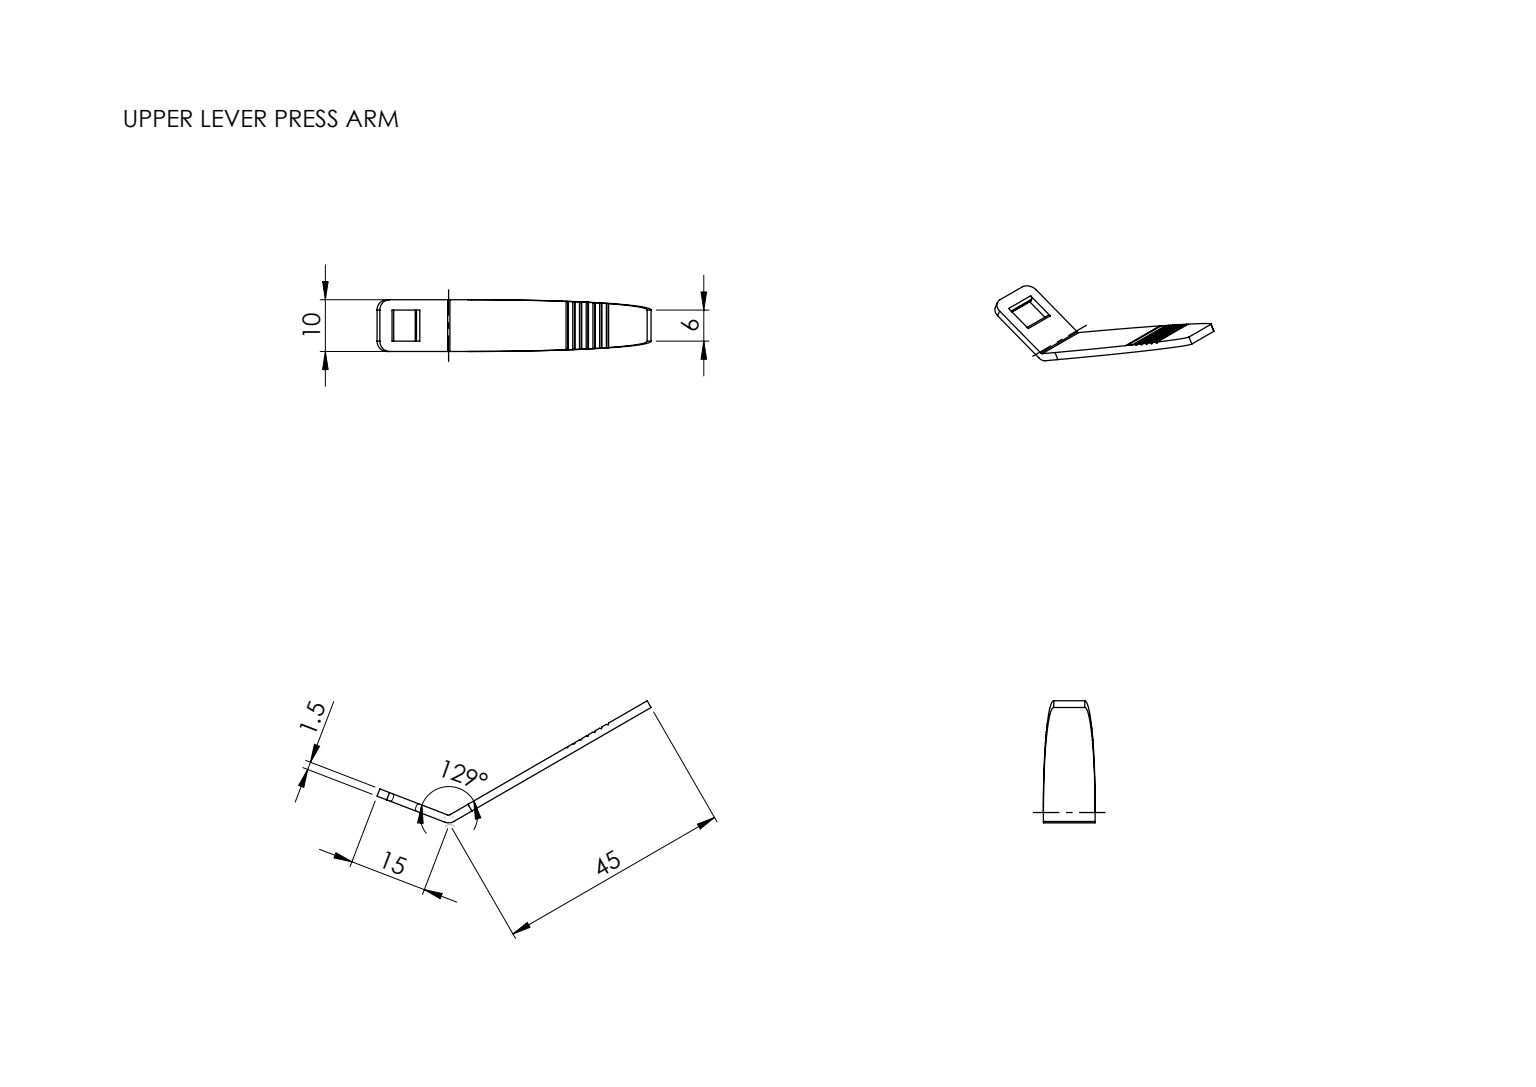
ISO-10303-21;
HEADER;
FILE_DESCRIPTION (('STEP AP214'),
    '1' );
FILE_NAME ('Upper Lever Press Arm.step',
    '2026-09-30T04:43:20',
    ( '' ),
    ( '' ),
    'SwSTEP 2.0',
    'SolidWorks 2026',
    '' );
FILE_SCHEMA (( 'AUTOMOTIVE_DESIGN' ));
ENDSEC;

DATA;
#3=B_SPLINE_CURVE_WITH_KNOTS ( 'NONE', 3,
 ( #22146, #34945, #44004, #5128 ),
 .UNSPECIFIED., .F., .F.,
 ( 4, 4 ),
 ( 1.885719144749635755E-05, 0.0003537736795864013565 ),
 .UNSPECIFIED. ) ;
#4=DIRECTION ( 'NONE',  ( 0.9659258262890682012, -0.2588190451025213501, 0.000000000000000000 ) ) ;
#132=CARTESIAN_POINT ( 'NONE',  ( -22.94165982901027689, 19.41290236794502277, -4.465504107374588472 ) ) ;
#193=CARTESIAN_POINT ( 'NONE',  ( -28.44450197225234334, 14.50378416766731959, -4.731833325462559969 ) ) ;
#237=LINE ( 'NONE', #8811, #24972 ) ;
#310=B_SPLINE_CURVE_WITH_KNOTS ( 'NONE', 3,
 ( #32716, #11134, #41787, #2878 ),
 .UNSPECIFIED., .F., .F.,
 ( 4, 4 ),
 ( 0.000000000000000000, 0.0003538863460372422966 ),
 .UNSPECIFIED. ) ;
#369=FACE_OUTER_BOUND ( 'NONE', #44588, .T. ) ;
#373=CARTESIAN_POINT ( 'NONE',  ( -27.13182931993292257, 16.99370688441070953, -4.657437592157545936 ) ) ;
#418=DIRECTION ( 'NONE',  ( -0.2588190451025176864, -0.9659258262890692004, 0.000000000000000000 ) ) ;
#455=EDGE_CURVE ( 'NONE', #37705, #6581, #56077, .T. ) ;
#460=VERTEX_POINT ( 'NONE', #2963 ) ;
#518=EDGE_CURVE ( 'NONE', #53934, #18987, #43004, .T. ) ;
#531=AXIS2_PLACEMENT_3D ( 'NONE', #51602, #12442, #13280 ) ;
#533=ADVANCED_FACE ( 'NONE', ( #51248 ), #3542, .F. ) ;
#534=AXIS2_PLACEMENT_3D ( 'NONE', #24826, #46384, #7499 ) ;
#571=AXIS2_PLACEMENT_3D ( 'NONE', #25411, #12058, #16909 ) ;
#582=( NAMED_UNIT ( * ) PLANE_ANGLE_UNIT ( ) SI_UNIT ( $, .RADIAN. ) );
#607=VERTEX_POINT ( 'NONE', #29699 ) ;
#614=ORIENTED_EDGE ( 'NONE', *, *, #13717, .F. ) ;
#616=VECTOR ( 'NONE', #50544, 1000.000000000000000 ) ;
#646=PLANE ( 'NONE',  #28564 ) ;
#675=DIRECTION ( 'NONE',  ( 0.2113248654051873565, 0.7886751345948123104, 0.5773502691896265082 ) ) ;
#682=VERTEX_POINT ( 'NONE', #21973 ) ;
#688=ORIENTED_EDGE ( 'NONE', *, *, #44373, .T. ) ;
#692=LINE ( 'NONE', #17737, #6878 ) ;
#697=CARTESIAN_POINT ( 'NONE',  ( -23.39689027546016220, 18.96061615304027370, 4.493364425890089109 ) ) ;
#727=EDGE_CURVE ( 'NONE', #44683, #32191, #692, .T. ) ;
#732=CARTESIAN_POINT ( 'NONE',  ( -16.70782865829815833, 23.01200647243835462, -4.019104856592038644 ) ) ;
#746=EDGE_CURVE ( 'NONE', #48518, #40704, #31739, .T. ) ;
#780=CARTESIAN_POINT ( 'NONE',  ( -20.79248460937205323, 18.92167845196996367, -4.386225263874957037 ) ) ;
#841=FILL_AREA_STYLE_COLOUR ( '', #31666 ) ;
#914=ORIENTED_EDGE ( 'NONE', *, *, #11163, .T. ) ;
#919=CARTESIAN_POINT ( 'NONE',  ( -50.99228148001754590, 2.341865487272627000, 5.000000000000000000 ) ) ;
#945=ORIENTED_EDGE ( 'NONE', *, *, #16723, .T. ) ;
#951=FILL_AREA_STYLE_COLOUR ( '', #1196 ) ;
#958=DIRECTION ( 'NONE',  ( 0.9335804264972041855, -0.3583679495452941621, 0.000000000000000000 ) ) ;
#963=EDGE_LOOP ( 'NONE', ( #48660, #54179, #26989, #34399, #45764, #5188, #19645, #55104, #36476, #32181 ) ) ;
#968=CARTESIAN_POINT ( 'NONE',  ( -21.06965149344186372, 20.49370688441071664, 4.356723378946029790 ) ) ;
#974=DIRECTION ( 'NONE',  ( 0.000000000000000000, 0.000000000000000000, 1.000000000000000000 ) ) ;
#985=CARTESIAN_POINT ( 'NONE',  ( -16.14528680376529834, 23.33679016358333769, -3.961395337094443914 ) ) ;
#1039=FACE_BOUND ( 'NONE', #10706, .T. ) ;
#1042=CARTESIAN_POINT ( 'NONE',  ( -28.39101450145270178, 14.53466517333176533, -4.730044803147324117 ) ) ;
#1050=CARTESIAN_POINT ( 'NONE',  ( -22.26155136248034694, 19.71499928042501537, 4.429874044484920503 ) ) ;
#1107=LINE ( 'NONE', #22455, #28687 ) ;
#1123=FACE_OUTER_BOUND ( 'NONE', #15703, .T. ) ;
#1180=ORIENTED_EDGE ( 'NONE', *, *, #37039, .T. ) ;
#1191=EDGE_LOOP ( 'NONE', ( #4345, #38872, #49783 ) ) ;
#1196=COLOUR_RGB ( '', 0.40784314, 0.44705882, 0.49803922) ;
#1254=DIRECTION ( 'NONE',  ( 0.9659258262890682012, -0.2588190451025213501, 0.000000000000000000 ) ) ;
#1307=LINE ( 'NONE', #53002, #19425 ) ;
#1330=CARTESIAN_POINT ( 'NONE',  ( -24.92324194630820244, 18.23204470015658174, -4.564397236248976419 ) ) ;
#1405=PRESENTATION_STYLE_ASSIGNMENT (( #23550 ) ) ;
#1409=CARTESIAN_POINT ( 'NONE',  ( -25.83279121425626812, 17.74370688441070953, -4.657437592157546824 ) ) ;
#1456=AXIS2_PLACEMENT_3D ( 'NONE', #26545, #39337, #35359 ) ;
#1459=DIRECTION ( 'NONE',  ( -0.9335804264972041855, 0.3583679495452941621, 0.000000000000000000 ) ) ;
#1498=AXIS2_PLACEMENT_3D ( 'NONE', #24554, #42170, #41870 ) ;
#1509=CIRCLE ( 'NONE', #36867, 0.5000000000000004441 ) ;
#1533=VECTOR ( 'NONE', #44302, 1000.000000000000114 ) ;
#1551=ORIENTED_EDGE ( 'NONE', *, *, #30791, .T. ) ;
#1552=EDGE_CURVE ( 'NONE', #19985, #6581, #39063, .T. ) ;
#1599=CARTESIAN_POINT ( 'NONE',  ( -27.56484202182514665, 16.74370688441070953, -4.657437592157546824 ) ) ;
#1634=CARTESIAN_POINT ( 'NONE',  ( -28.32679246876683266, 14.57174378119085389, 4.727889153708476400 ) ) ;
#1636=LINE ( 'NONE', #18963, #55409 ) ;
#1736=CARTESIAN_POINT ( 'NONE',  ( -56.02165185617580079, 5.343604887189308705, 2.999999999999993339 ) ) ;
#1741=B_SPLINE_CURVE_WITH_KNOTS ( 'NONE', 3,
 ( #23369, #39838, #22787, #52607 ),
 .UNSPECIFIED., .F., .F.,
 ( 4, 4 ),
 ( 0.0001251225081293656771, 0.0003537265380804738486 ),
 .UNSPECIFIED. ) ;
#1743=PLANE ( 'NONE',  #41578 ) ;
#1765=DIRECTION ( 'NONE',  ( -1.007958083594381669E-15, 3.869188571150967118E-16, -1.000000000000000000 ) ) ;
#1827=CARTESIAN_POINT ( 'NONE',  ( -20.11552963796318494, 21.04456939451101150, -4.294601649057681492 ) ) ;
#1840=CARTESIAN_POINT ( 'NONE',  ( -29.14071270714143935, 15.83387752003526394, 4.730034822273776030 ) ) ;
#1943=CARTESIAN_POINT ( 'NONE',  ( -11.88054826722768276, 25.79903810567671130, 3.000000000000000888 ) ) ;
#1988=CARTESIAN_POINT ( 'NONE',  ( -11.88054826722768276, 25.79903810567671130, 5.000000000000000000 ) ) ;
#2121=CARTESIAN_POINT ( 'NONE',  ( -29.26563357085082728, 15.76175442574525043, 4.734210823084358921 ) ) ;
#2142=VERTEX_POINT ( 'NONE', #17518 ) ;
#2186=ORIENTED_EDGE ( 'NONE', *, *, #25414, .T. ) ;
#2193=VECTOR ( 'NONE', #958, 999.9999999999998863 ) ;
#2213=CARTESIAN_POINT ( 'NONE',  ( -46.28406441860501985, 5.387676038879166462, 5.000000000000000000 ) ) ;
#2217=ORIENTED_EDGE ( 'NONE', *, *, #55126, .F. ) ;
#2296=PLANE ( 'NONE',  #21068 ) ;
#2410=DIRECTION ( 'NONE',  ( 0.3583679495452941066, 0.9335804264972041855, -0.000000000000000000 ) ) ;
#2412=CARTESIAN_POINT ( 'NONE',  ( -22.03063064900203827, 19.66612883677992585, 4.421226519471689542 ) ) ;
#2427=ORIENTED_EDGE ( 'NONE', *, *, #28275, .F. ) ;
#2432=AXIS2_PLACEMENT_3D ( 'NONE', #47385, #8496, #54174 ) ;
#2450=CARTESIAN_POINT ( 'NONE',  ( -27.13299098042555002, 16.99303619941258603, -4.657414165320978405 ) ) ;
#2462=CARTESIAN_POINT ( 'NONE',  ( -23.66772770479517618, 18.99370688441070953, -4.503111145262439052 ) ) ;
#2485=ORIENTED_EDGE ( 'NONE', *, *, #28912, .F. ) ;
#2568=FACE_OUTER_BOUND ( 'NONE', #32711, .T. ) ;
#2573=CARTESIAN_POINT ( 'NONE',  ( -58.57533928340691887, 0.08623575067603483912, 2.999999999999993339 ) ) ;
#2604=ORIENTED_EDGE ( 'NONE', *, *, #55126, .T. ) ;
#2610=AXIS2_PLACEMENT_3D ( 'NONE', #34638, #13373, #3697 ) ;
#2628=DIRECTION ( 'NONE',  ( -0.000000000000000000, -0.000000000000000000, 1.000000000000000000 ) ) ;
#2637=CARTESIAN_POINT ( 'NONE',  ( -22.02230666951336246, 19.67040017278726438, 4.420763615217817133 ) ) ;
#2683=EDGE_LOOP ( 'NONE', ( #55117, #19603, #53392, #16395 ) ) ;
#2686=ORIENTED_EDGE ( 'NONE', *, *, #5710, .F. ) ;
#2691=PLANE ( 'NONE',  #38679 ) ;
#2713=ORIENTED_EDGE ( 'NONE', *, *, #38351, .F. ) ;
#2763=CARTESIAN_POINT ( 'NONE',  ( -19.33760068587298164, 21.49370688441072019, 4.239878526350478793 ) ) ;
#2766=DIRECTION ( 'NONE',  ( 0.3535533905932738974, -0.6123724356957929160, -0.7071067811865487940 ) ) ;
#2785=EDGE_LOOP ( 'NONE', ( #40511, #29941, #51061 ) ) ;
#2800=( BOUNDED_SURFACE ( )  B_SPLINE_SURFACE ( 2, 3, ( 
 ( #15547, #23270, #2213, #41672 ),
 ( #28335, #15020, #45653, #32877 ),
 ( #27817, #11304, #28636, #40593 ) ),
 .UNSPECIFIED., .F., .F., .T. ) 
 B_SPLINE_SURFACE_WITH_KNOTS ( ( 3, 3 ),
 ( 4, 4 ),
 ( 0.000000000000000000, 1.000000000000000000 ),
 ( -0.001575000000000004998, 7.500000000001961749E-05 ),
 .UNSPECIFIED. ) 
 GEOMETRIC_REPRESENTATION_ITEM ( )  RATIONAL_B_SPLINE_SURFACE ( (
 ( 1.000000000000000000, 1.000000000000000000, 1.000000000000000000, 1.000000000000000000),
 ( 0.7071067811865475727, 0.7071067811865475727, 0.7071067811865484609, 0.7071067811865484609),
 ( 1.000000000000000000, 1.000000000000000000, 1.000000000000000000, 1.000000000000000000) ) ) 
 REPRESENTATION_ITEM ( '' )  SURFACE ( )  );
#2812=DIRECTION ( 'NONE',  ( 0.9659258262890692004, -0.2588190451025176864, 0.000000000000000000 ) ) ;
#2829=DIRECTION ( 'NONE',  ( 0.9335804264972041855, -0.3583679495452941066, 0.000000000000000000 ) ) ;
#2855=EDGE_CURVE ( 'NONE', #53976, #35993, #43666, .T. ) ;
#2878=CARTESIAN_POINT ( 'NONE',  ( -19.77061338776520216, 21.24370688441071664, -4.270683379717145733 ) ) ;
#2911=VERTEX_POINT ( 'NONE', #46208 ) ;
#2944=CARTESIAN_POINT ( 'NONE',  ( -46.00906441860537655, 4.911362066797487103, -5.000000000000000000 ) ) ;
#2963=CARTESIAN_POINT ( 'NONE',  ( -60.92294909528611413, 7.225036622302098976, 2.999999999999993339 ) ) ;
#3005=CARTESIAN_POINT ( 'NONE',  ( -23.66772770479517618, 18.99370688441070953, -4.657437592157546824 ) ) ;
#3035=B_SPLINE_CURVE_WITH_KNOTS ( 'NONE', 3,
 ( #45030, #32522, #1827, #23445, #5547, #44723, #19152, #41320, #36223, #23165, #36482 ),
 .UNSPECIFIED., .F., .F.,
 ( 4, 1, 1, 2, 2, 1, 4 ),
 ( 0.2333392773190904879, 0.2451180778799246229, 0.2480627780201330179, 0.2495351280902372015, 0.2502713031252893350, 0.2510074781603415239, 0.2568968784407584804 ),
 .UNSPECIFIED. ) ;
#3158=CARTESIAN_POINT ( 'NONE',  ( -63.00984630926863161, 1.788483511016180305, 2.999999999999993339 ) ) ;
#3275=ADVANCED_FACE ( 'NONE', ( #21789 ), #18361, .F. ) ;
#3318=CARTESIAN_POINT ( 'NONE',  ( -13.01064681732981398, 25.14657540356444088, -3.506683753893632183 ) ) ;
#3363=DIRECTION ( 'NONE',  ( -0.7886751345948130876, 0.2113248654051844977, 0.5773502691896263972 ) ) ;
#3375=DIRECTION ( 'NONE',  ( 0.9659258262890692004, -0.2588190451025176864, 0.000000000000000000 ) ) ;
#3426=ORIENTED_EDGE ( 'NONE', *, *, #37039, .F. ) ;
#3434=CARTESIAN_POINT ( 'NONE',  ( -22.02230563637845151, 19.67040402849924163, -4.420763475398227449 ) ) ;
#3449=B_SPLINE_CURVE_WITH_KNOTS ( 'NONE', 3,
 ( #47504, #55745, #16551, #4070 ),
 .UNSPECIFIED., .F., .F.,
 ( 4, 4 ),
 ( 0.0001648889278767292786, 0.0003345323828099543780 ),
 .UNSPECIFIED. ) ;
#3450=CARTESIAN_POINT ( 'NONE',  ( -21.93567689722629765, 19.99370688441071309, -4.657437592157546824 ) ) ;
#3452=CARTESIAN_POINT ( 'NONE',  ( -26.26580391614848864, 17.49370688441070953, -4.622528711259356271 ) ) ;
#3464=EDGE_LOOP ( 'NONE', ( #10205, #16971, #45019 ) ) ;
#3503=CARTESIAN_POINT ( 'NONE',  ( -60.88973930853472183, 7.404220597074750110, 2.999999999999993339 ) ) ;
#3513=VERTEX_POINT ( 'NONE', #55810 ) ;
#3528=CARTESIAN_POINT ( 'NONE',  ( -11.91804826722769128, 25.86399001096056338, -3.000000000000000000 ) ) ;
#3529=CYLINDRICAL_SURFACE ( 'NONE', #534, 0.5000000000000004441 ) ;
#3540=CARTESIAN_POINT ( 'NONE',  ( -13.18266667305592499, 23.31520888598613084, -3.678144203997483430 ) ) ;
#3542=PLANE ( 'NONE',  #47657 ) ;
#3622=DIRECTION ( 'NONE',  ( -0.000000000000000000, -0.000000000000000000, -1.000000000000000000 ) ) ;
#3675=CARTESIAN_POINT ( 'NONE',  ( -25.85160320928759248, 17.67349956316208193, 4.606045228336897779 ) ) ;
#3697=DIRECTION ( 'NONE',  ( 1.000000000000000000, 0.000000000000000000, 0.000000000000000000 ) ) ;
#3709=ORIENTED_EDGE ( 'NONE', *, *, #38832, .F. ) ;
#3718=EDGE_CURVE ( 'NONE', #18779, #46324, #15132, .T. ) ;
#3727=PLANE ( 'NONE',  #24862 ) ;
#3739=ORIENTED_EDGE ( 'NONE', *, *, #43733, .F. ) ;
#3749=PLANE ( 'NONE',  #37824 ) ;
#3752=VERTEX_POINT ( 'NONE', #14884 ) ;
#3823=DIRECTION ( 'NONE',  ( 0.9659258262890682012, -0.2588190451025213501, 0.000000000000000000 ) ) ;
#3848=CARTESIAN_POINT ( 'NONE',  ( -20.16419826038267260, 21.01647055225602401, 4.297939206181997207 ) ) ;
#3851=CARTESIAN_POINT ( 'NONE',  ( -22.02230563637845151, 19.67040402849924163, -4.420763475398227449 ) ) ;
#3858=CARTESIAN_POINT ( 'NONE',  ( -50.45472955569960760, 3.742236127018431890, 5.000000000000000000 ) ) ;
#3887=EDGE_LOOP ( 'NONE', ( #8947, #2217, #37332, #24607 ) ) ;
#3889=ORIENTED_EDGE ( 'NONE', *, *, #36503, .T. ) ;
#3924=LINE ( 'NONE', #52478, #14635 ) ;
#3952=AXIS2_PLACEMENT_3D ( 'NONE', #17630, #4, #38360 ) ;
#3976=ADVANCED_FACE ( 'NONE', ( #56031, #44080 ), #646, .T. ) ;
#3981=DIRECTION ( 'NONE',  ( 1.007958083594381472E-15, -3.869188571150966132E-16, 1.000000000000000000 ) ) ;
#4011=EDGE_LOOP ( 'NONE', ( #28267, #55445, #12491, #53597 ) ) ;
#4044=ORIENTED_EDGE ( 'NONE', *, *, #50823, .F. ) ;
#4066=ORIENTED_EDGE ( 'NONE', *, *, #49513, .F. ) ;
#4070=CARTESIAN_POINT ( 'NONE',  ( -23.29661890453421691, 19.01267837833611551, -4.488312987714206059 ) ) ;
#4092=VERTEX_POINT ( 'NONE', #3434 ) ;
#4123=PLANE ( 'NONE',  #571 ) ;
#4149=CARTESIAN_POINT ( 'NONE',  ( -22.65299646082626239, 19.57956224127125111, 4.449815307286153043 ) ) ;
#4195=ORIENTED_EDGE ( 'NONE', *, *, #45589, .T. ) ;
#4222=CARTESIAN_POINT ( 'NONE',  ( -21.06965149344186372, 20.49370688441071664, -4.356725136697556344 ) ) ;
#4233=CARTESIAN_POINT ( 'NONE',  ( -19.63965433603666710, 19.58726532061008641, 4.312915315567922292 ) ) ;
#4238=CARTESIAN_POINT ( 'NONE',  ( -61.10213307005876970, 6.758246409053502823, -3.000000000000006217 ) ) ;
#4300=AXIS2_PLACEMENT_3D ( 'NONE', #38438, #30777, #26785 ) ;
#4345=ORIENTED_EDGE ( 'NONE', *, *, #55262, .F. ) ;
#4354=CARTESIAN_POINT ( 'NONE',  ( -20.72814514249575168, 20.40220053346460460, -4.343046601173932153 ) ) ;
#4360=EDGE_LOOP ( 'NONE', ( #51718, #33979, #28900, #15955 ) ) ;
#4382=PLANE ( 'NONE',  #4300 ) ;
#4399=CARTESIAN_POINT ( 'NONE',  ( -15.36885972723471561, 22.05300973765551475, -3.958603441819915414 ) ) ;
#4487=CARTESIAN_POINT ( 'NONE',  ( -19.77061338776520216, 21.24370688441071664, -4.657437592157546824 ) ) ;
#4490=CARTESIAN_POINT ( 'NONE',  ( -19.70957090889394081, 19.54689896845012598, -4.317539206161682408 ) ) ;
#4495=VERTEX_POINT ( 'NONE', #37008 ) ;
#4496=CARTESIAN_POINT ( 'NONE',  ( -19.52344721837093999, 19.65435753127615470, 4.305181340342182139 ) ) ;
#4499=EDGE_CURVE ( 'NONE', #19187, #9690, #14862, .T. ) ;
#4529=ORIENTED_EDGE ( 'NONE', *, *, #8617, .F. ) ;
#4537=CARTESIAN_POINT ( 'NONE',  ( -62.23823698199103660, 6.658783344088820222, -3.000000000000000000 ) ) ;
#4543=EDGE_CURVE ( 'NONE', #19187, #51242, #19685, .T. ) ;
#4555=CARTESIAN_POINT ( 'NONE',  ( -24.53374897521541698, 18.49370927080960669, -4.545578601930409413 ) ) ;
#4628=ORIENTED_EDGE ( 'NONE', *, *, #18960, .F. ) ;
#4629=CARTESIAN_POINT ( 'NONE',  ( -56.66762604419704985, 5.055998648713356580, -3.000000000000007105 ) ) ;
#4630=CARTESIAN_POINT ( 'NONE',  ( -24.74851972188836058, 18.25476655873277920, 4.557895469182953185 ) ) ;
#4701=CARTESIAN_POINT ( 'NONE',  ( -22.04728230093569152, 19.65758605842115969, -4.422151119964278010 ) ) ;
#4708=CARTESIAN_POINT ( 'NONE',  ( -63.56784591066751489, 8.775889882925216767, 5.000000000000000000 ) ) ;
#4759=CARTESIAN_POINT ( 'NONE',  ( -19.95056665410288943, 19.40776001008019236, -4.333296610429257179 ) ) ;
#4791=ORIENTED_EDGE ( 'NONE', *, *, #38882, .F. ) ;
#4839=EDGE_CURVE ( 'NONE', #27103, #49013, #33304, .T. ) ;
#4852=EDGE_LOOP ( 'NONE', ( #39303, #3889, #32640 ) ) ;
#4945=ADVANCED_FACE ( 'NONE', ( #23385 ), #17999, .F. ) ;
#4973=DIRECTION ( 'NONE',  ( 0.9659258262890692004, -0.2588190451025176864, 0.000000000000000000 ) ) ;
#5001=( BOUNDED_CURVE ( )  B_SPLINE_CURVE ( 2, ( #41086, #22935, #10981 ),
 .UNSPECIFIED., .F., .F. ) 
 B_SPLINE_CURVE_WITH_KNOTS ( ( 3, 3 ),
 ( 0.6158339227882835276, 0.6249778499672641319 ),
 .UNSPECIFIED. ) 
 CURVE ( )  GEOMETRIC_REPRESENTATION_ITEM ( )  RATIONAL_B_SPLINE_CURVE ( ( 0.8614131787543850560, 0.8620336302495723579, 0.8627030601714029689 ) ) 
 REPRESENTATION_ITEM ( '' )  );
#5045=CIRCLE ( 'NONE', #15888, 0.5000000000000004441 ) ;
#5058=CARTESIAN_POINT ( 'NONE',  ( -37.15891100857655971, 9.472517764717013122, -4.937199669358084186 ) ) ;
#5085=VECTOR ( 'NONE', #43649, 1000.000000000000114 ) ;
#5086=EDGE_LOOP ( 'NONE', ( #37843, #20900, #27083, #46358, #51235, #17479, #25512 ) ) ;
#5115=FACE_OUTER_BOUND ( 'NONE', #17806, .T. ) ;
#5128=CARTESIAN_POINT ( 'NONE',  ( -21.93567466420777379, 19.99370817364452790, -4.408991681665293427 ) ) ;
#5188=ORIENTED_EDGE ( 'NONE', *, *, #50318, .T. ) ;
#5193=DIRECTION ( 'NONE',  ( -1.000000000000000000, 0.000000000000000000, 0.000000000000000000 ) ) ;
#5233=ADVANCED_FACE ( 'NONE', ( #46610 ), #3727, .F. ) ;
#5265=DIRECTION ( 'NONE',  ( -1.000000000000000000, 0.000000000000000000, 0.000000000000000000 ) ) ;
#5275=CARTESIAN_POINT ( 'NONE',  ( -56.20083583094844926, 4.876814673940706335, 2.999999999999993339 ) ) ;
#5307=CARTESIAN_POINT ( 'NONE',  ( -19.42910703681909368, 21.15220053346460816, -4.255330291692488665 ) ) ;
#5338=CARTESIAN_POINT ( 'NONE',  ( -19.68509517508318751, 19.56103003995438883, -4.315923200200658449 ) ) ;
#5382=ORIENTED_EDGE ( 'NONE', *, *, #29011, .T. ) ;
#5388=ORIENTED_EDGE ( 'NONE', *, *, #28680, .F. ) ;
#5398=( NAMED_UNIT ( * ) SI_UNIT ( $, .STERADIAN. ) SOLID_ANGLE_UNIT ( ) );
#5452=VECTOR ( 'NONE', #49321, 1000.000000000000114 ) ;
#5543=CARTESIAN_POINT ( 'NONE',  ( -14.23203706048740713, 24.44140541789180787, -3.724779944465314241 ) ) ;
#5547=CARTESIAN_POINT ( 'NONE',  ( -20.39013098992649020, 20.88602823003513365, -4.312947112340340006 ) ) ;
#5560=CARTESIAN_POINT ( 'NONE',  ( -38.30474801573077315, 10.54301926775796439, 4.960515765732081306 ) ) ;
#5561=ORIENTED_EDGE ( 'NONE', *, *, #53550, .F. ) ;
#5569=ORIENTED_EDGE ( 'NONE', *, *, #23443, .F. ) ;
#5591=ORIENTED_EDGE ( 'NONE', *, *, #52151, .F. ) ;
#5604=CARTESIAN_POINT ( 'NONE',  ( -45.77156441860526570, 4.499999999999973355, 5.000000000000000000 ) ) ;
#5663=( NAMED_UNIT ( * ) SI_UNIT ( $, .STERADIAN. ) SOLID_ANGLE_UNIT ( ) );
#5695=EDGE_CURVE ( 'NONE', #35896, #40396, #13626, .T. ) ;
#5696=VECTOR ( 'NONE', #40835, 1000.000000000000000 ) ;
#5710=EDGE_CURVE ( 'NONE', #35896, #41243, #40512, .T. ) ;
#5711=EDGE_CURVE ( 'NONE', #54087, #19187, #10399, .T. ) ;
#5730=VECTOR ( 'NONE', #40205, 1000.000000000000000 ) ;
#5732=CARTESIAN_POINT ( 'NONE',  ( -50.02554558092695913, 3.776013638374817294, 5.000000000000000000 ) ) ;
#5807=DIRECTION ( 'NONE',  ( 0.3535533905932752297, -0.6123724356957952475, -0.7071067811865462405 ) ) ;
#5809=VECTOR ( 'NONE', #41899, 1000.000000000000000 ) ;
#5816=CARTESIAN_POINT ( 'NONE',  ( -27.13299098042555002, 16.99303619941258603, -4.657414165320978405 ) ) ;
#5838=CARTESIAN_POINT ( 'NONE',  ( -13.83440620147302269, 24.67097770138186874, -3.662372917584403087 ) ) ;
#5862=ORIENTED_EDGE ( 'NONE', *, *, #37251, .T. ) ;
#5864=ORIENTED_EDGE ( 'NONE', *, *, #50563, .T. ) ;
#5918=VERTEX_POINT ( 'NONE', #6685 ) ;
#5926=EDGE_CURVE ( 'NONE', #18779, #21631, #8828, .T. ) ;
#5927=CARTESIAN_POINT ( 'NONE',  ( -56.38001980572109062, 4.410024460692103077, -3.000000000000007105 ) ) ;
#5949=CARTESIAN_POINT ( 'NONE',  ( -61.38973930853472183, 7.404220597074748333, 2.999999999999993339 ) ) ;
#5959=CARTESIAN_POINT ( 'NONE',  ( -20.72814514249575168, 20.40220053346460460, 4.343046601168861542 ) ) ;
#5964=LINE ( 'NONE', #49096, #29767 ) ;
#5968=( NAMED_UNIT ( * ) PLANE_ANGLE_UNIT ( ) SI_UNIT ( $, .RADIAN. ) );
#5976=CIRCLE ( 'NONE', #11382, 0.5000000000000004441 ) ;
#5983=VECTOR ( 'NONE', #42987, 1000.000000000000000 ) ;
#6085=CARTESIAN_POINT ( 'NONE',  ( -50.27554558092695913, 4.209026340267034705, 5.000000000000000000 ) ) ;
#6091=DIRECTION ( 'NONE',  ( -0.000000000000000000, -0.000000000000000000, 1.000000000000000000 ) ) ;
#6101=CARTESIAN_POINT ( 'NONE',  ( -21.06965149344186372, 20.49370688441071664, -4.657437592157546824 ) ) ;
#6116=CARTESIAN_POINT ( 'NONE',  ( -61.21055533376208757, 7.871010810323348039, -3.000000000000007105 ) ) ;
#6117=ORIENTED_EDGE ( 'NONE', *, *, #50563, .F. ) ;
#6154=CARTESIAN_POINT ( 'NONE',  ( -30.55480944230645690, 15.01744838932757276, 4.775844711708173485 ) ) ;
#6263=B_SPLINE_CURVE_WITH_KNOTS ( 'NONE', 3,
 ( #10723, #10967, #1330, #28286 ),
 .UNSPECIFIED., .F., .F.,
 ( 4, 4 ),
 ( 0.0002184642560491729404, 0.0003536952807433174899 ),
 .UNSPECIFIED. ) ;
#6321=ADVANCED_FACE ( 'NONE', ( #8876 ), #21359, .T. ) ;
#6376=DIRECTION ( 'NONE',  ( -0.9335804264972041855, 0.3583679495452941621, 0.000000000000000000 ) ) ;
#6432=PRODUCT_DEFINITION_CONTEXT ( 'detailed design', #56163, 'design' ) ;
#6435=CARTESIAN_POINT ( 'NONE',  ( -44.89558674184503673, 6.737796755050466935, -5.000000000000005329 ) ) ;
#6494=PLANE ( 'NONE',  #45542 ) ;
#6505=CARTESIAN_POINT ( 'NONE',  ( -11.38054826722768098, 24.93301270189227381, 3.000000000000000000 ) ) ;
#6535=ORIENTED_EDGE ( 'NONE', *, *, #19165, .T. ) ;
#6580=ORIENTED_EDGE ( 'NONE', *, *, #52151, .T. ) ;
#6581=VERTEX_POINT ( 'NONE', #19313 ) ;
#6589=CARTESIAN_POINT ( 'NONE',  ( -19.42910703681909368, 21.15220053346460816, 4.255330291687501543 ) ) ;
#6683=EDGE_LOOP ( 'NONE', ( #33292, #29988, #10668, #9770 ) ) ;
#6685=CARTESIAN_POINT ( 'NONE',  ( -61.74810725808002587, 6.470640170577546257, -3.000000000000007105 ) ) ;
#6689=ORIENTED_EDGE ( 'NONE', *, *, #33111, .T. ) ;
#6723=ORIENTED_EDGE ( 'NONE', *, *, #19766, .F. ) ;
#6817=AXIS2_PLACEMENT_3D ( 'NONE', #16793, #12546, #20187 ) ;
#6825=VERTEX_POINT ( 'NONE', #39738 ) ;
#6832=ORIENTED_EDGE ( 'NONE', *, *, #727, .T. ) ;
#6857=ADVANCED_FACE ( 'NONE', ( #9915 ), #31196, .T. ) ;
#6878=VECTOR ( 'NONE', #31053, 1000.000000000000114 ) ;
#6887=CARTESIAN_POINT ( 'NONE',  ( -19.36810218178846910, 21.37987375194729367, 4.244941833917287077 ) ) ;
#6896=DIRECTION ( 'NONE',  ( -0.000000000000000000, -0.000000000000000000, 1.000000000000000000 ) ) ;
#7026=AXIS2_PLACEMENT_3D ( 'NONE', #8681, #20618, #43325 ) ;
#7058=AXIS2_PLACEMENT_3D ( 'NONE', #5732, #13433, #18217 ) ;
#7154=EDGE_CURVE ( 'NONE', #21504, #10403, #14203, .T. ) ;
#7177=ORIENTED_EDGE ( 'NONE', *, *, #11568, .F. ) ;
#7189=CARTESIAN_POINT ( 'NONE',  ( -26.26580391614848864, 17.49370688441070953, -4.657437592157546824 ) ) ;
#7222=ORIENTED_EDGE ( 'NONE', *, *, #55454, .T. ) ;
#7274=VERTEX_POINT ( 'NONE', #42088 ) ;
#7283=CARTESIAN_POINT ( 'NONE',  ( -22.02230666951336246, 19.67040017278726438, 4.420763615217817133 ) ) ;
#7361=AXIS2_PLACEMENT_3D ( 'NONE', #26935, #51898, #13017 ) ;
#7388=CARTESIAN_POINT ( 'NONE',  ( -11.88054826722768276, 25.79903810567671130, -3.000000000000000000 ) ) ;
#7435=ORIENTED_EDGE ( 'NONE', *, *, #7154, .F. ) ;
#7444=EDGE_CURVE ( 'NONE', #6825, #29855, #42683, .T. ) ;
#7499=DIRECTION ( 'NONE',  ( 1.000000000000000000, 0.000000000000000000, -8.673617379884027583E-16 ) ) ;
#7555=CARTESIAN_POINT ( 'NONE',  ( -20.53083501583961734, 20.80479272279814040, 4.322231945293713906 ) ) ;
#7556=CARTESIAN_POINT ( 'NONE',  ( -26.24927669643210848, 17.48927842923457021, -4.622014950999592031 ) ) ;
#7561=CARTESIAN_POINT ( 'NONE',  ( -13.00144731260268038, 25.15188674009506542, -3.504651694023052766 ) ) ;
#7567=DIRECTION ( 'NONE',  ( -0.9335804264972042965, 0.3583679495452938291, -0.000000000000000000 ) ) ;
#7592=CARTESIAN_POINT ( 'NONE',  ( -24.96676581047183063, 18.24370688441070953, -4.565775476651154463 ) ) ;
#7604=CARTESIAN_POINT ( 'NONE',  ( -23.44005680416443838, 18.93270265044663603, 4.490773887887535842 ) ) ;
#7659=VERTEX_POINT ( 'NONE', #14520 ) ;
#7677=DIRECTION ( 'NONE',  ( 0.000000000000000000, 0.000000000000000000, 1.000000000000000000 ) ) ;
#7729=B_SPLINE_CURVE_WITH_KNOTS ( 'NONE', 3,
 ( #49222, #10335, #27661, #44987 ),
 .UNSPECIFIED., .F., .F.,
 ( 4, 4 ),
 ( 0.7012410636449952772, 0.7288427234739881522 ),
 .UNSPECIFIED. ) ;
#7832=CARTESIAN_POINT ( 'NONE',  ( -19.42910703681909368, 21.15220053346460816, 4.255330291687501543 ) ) ;
#7915=LINE ( 'NONE', #7604, #47445 ) ;
#8073=LINE ( 'NONE', #16876, #21275 ) ;
#8135=CARTESIAN_POINT ( 'NONE',  ( -11.88054826722768276, 25.79903810567671130, -3.000000000000000000 ) ) ;
#8172=DIRECTION ( 'NONE',  ( -1.000000000000000000, 0.000000000000000000, 0.000000000000000000 ) ) ;
#8256=DIRECTION ( 'NONE',  ( 0.000000000000000000, 0.000000000000000000, -1.000000000000000000 ) ) ;
#8266=ORIENTED_EDGE ( 'NONE', *, *, #44650, .T. ) ;
#8284=ORIENTED_EDGE ( 'NONE', *, *, #40489, .T. ) ;
#8296=B_SPLINE_CURVE_WITH_KNOTS ( 'NONE', 3,
 ( #11566, #28883, #46181, #7283 ),
 .UNSPECIFIED., .F., .F.,
 ( 4, 4 ),
 ( 0.000000000000000000, 0.0003349204823136315776 ),
 .UNSPECIFIED. ) ;
#8325=EDGE_LOOP ( 'NONE', ( #15393, #45057, #35257, #5569 ) ) ;
#8375=FACE_OUTER_BOUND ( 'NONE', #29807, .T. ) ;
#8466=CARTESIAN_POINT ( 'NONE',  ( -19.36956794502930634, 19.74319977116263303, 4.294846203288412489 ) ) ;
#8496=DIRECTION ( 'NONE',  ( 0.9659258262890682012, -0.2588190451025213501, 0.000000000000000000 ) ) ;
#8504=CARTESIAN_POINT ( 'NONE',  ( -49.27554558092695913, 2.476975532698160620, 5.000000000000000000 ) ) ;
#8555=EDGE_LOOP ( 'NONE', ( #54942, #44710, #47319, #46606, #24688, #25642, #25519, #9963, #53675, #22278, #47759, #29937, #5388, #20429, #42126, #40703, #32041, #55171, #55584, #5591, #31627, #32561, #27281, #4628, #12436, #50794, #27262 ) ) ;
#8563=ORIENTED_EDGE ( 'NONE', *, *, #21234, .F. ) ;
#8564=ORIENTED_EDGE ( 'NONE', *, *, #50679, .F. ) ;
#8612=LINE ( 'NONE', #25944, #18397 ) ;
#8617=EDGE_CURVE ( 'NONE', #29855, #9917, #27180, .T. ) ;
#8642=CARTESIAN_POINT ( 'NONE',  ( -25.83279121425626812, 17.74370688441070953, 4.657440554554202805 ) ) ;
#8658=CARTESIAN_POINT ( 'NONE',  ( -13.19204130227259952, 23.30979644128433748, -3.679643887444146610 ) ) ;
#8674=EDGE_CURVE ( 'NONE', #50858, #45180, #46535, .T. ) ;
#8681=CARTESIAN_POINT ( 'NONE',  ( -62.23823698199103660, 6.658783344088824663, 3.000000000000000000 ) ) ;
#8706=CARTESIAN_POINT ( 'NONE',  ( -22.65298538027628794, 19.57956863862976249, -4.449819841089008854 ) ) ;
#8797=ORIENTED_EDGE ( 'NONE', *, *, #45589, .F. ) ;
#8811=CARTESIAN_POINT ( 'NONE',  ( -19.33760068587298164, 21.49370688441072019, -4.657437592157546824 ) ) ;
#8818=AXIS2_PLACEMENT_3D ( 'NONE', #16839, #43691, #35213 ) ;
#8819=CARTESIAN_POINT ( 'NONE',  ( -25.85160320928759248, 17.67349956316208193, 4.606045228336897779 ) ) ;
#8821=VECTOR ( 'NONE', #31799, 1000.000000000000000 ) ;
#8828=B_SPLINE_CURVE_WITH_KNOTS ( 'NONE', 3,
 ( #45864, #37071, #54372, #34757 ),
 .UNSPECIFIED., .F., .F.,
 ( 4, 4 ),
 ( 0.6233793831165909127, 0.6485820559972910182 ),
 .UNSPECIFIED. ) ;
#8876=FACE_OUTER_BOUND ( 'NONE', #32982, .T. ) ;
#8905=CARTESIAN_POINT ( 'NONE',  ( -26.21622229497770817, 17.48042152905857449, -4.621141326338904065 ) ) ;
#8927=DIRECTION ( 'NONE',  ( 0.8660254037844380415, 0.5000000000000011102, 0.000000000000000000 ) ) ;
#8928=ORIENTED_EDGE ( 'NONE', *, *, #29439, .T. ) ;
#8940=ORIENTED_EDGE ( 'NONE', *, *, #18960, .T. ) ;
#8941=CARTESIAN_POINT ( 'NONE',  ( -12.68893542602017988, 23.60026475436954740, -3.594889907554657427 ) ) ;
#8943=EDGE_LOOP ( 'NONE', ( #40478, #26337, #29664, #33700 ) ) ;
#8947=ORIENTED_EDGE ( 'NONE', *, *, #37432, .T. ) ;
#8963=ORIENTED_EDGE ( 'NONE', *, *, #33272, .T. ) ;
#8965=CARTESIAN_POINT ( 'NONE',  ( -56.20083583094844926, 4.876814673940706335, 2.999999999999993339 ) ) ;
#8969=CARTESIAN_POINT ( 'NONE',  ( -64.10539783498545319, 7.375519243179410545, 3.000000000000000000 ) ) ;
#8982=CARTESIAN_POINT ( 'NONE',  ( -45.77156441860526570, 4.499999999999973355, 5.000000000000000000 ) ) ;
#8983=CARTESIAN_POINT ( 'NONE',  ( -13.01702680972596227, 25.14289191323709360, -3.508089884283071669 ) ) ;
#8990=ORIENTED_EDGE ( 'NONE', *, *, #37009, .T. ) ;
#8991=CARTESIAN_POINT ( 'NONE',  ( -21.64218843024125860, 20.16315252982854034, -4.391944182239861050 ) ) ;
#8999=ORIENTED_EDGE ( 'NONE', *, *, #26082, .F. ) ;
#9021=DIRECTION ( 'NONE',  ( 0.000000000000000000, 0.000000000000000000, 1.000000000000000000 ) ) ;
#9051=ORIENTED_EDGE ( 'NONE', *, *, #19766, .T. ) ;
#9063=CARTESIAN_POINT ( 'NONE',  ( -50.27554558092695913, 4.209026340267034705, 5.000000000000000000 ) ) ;
#9082=CARTESIAN_POINT ( 'NONE',  ( -61.56892328330737030, 6.937430383826147740, 2.999999999999993339 ) ) ;
#9084=DIRECTION ( 'NONE',  ( 0.3535533905932738974, -0.6123724356957929160, -0.7071067811865487940 ) ) ;
#9115=CARTESIAN_POINT ( 'NONE',  ( -27.56460882755735398, 16.74384151918395247, 4.673983433494172779 ) ) ;
#9143=FACE_OUTER_BOUND ( 'NONE', #13193, .T. ) ;
#9171=CARTESIAN_POINT ( 'NONE',  ( -11.63054826722768453, 25.36602540378449788, -3.000000000000000000 ) ) ;
#9175=ORIENTED_EDGE ( 'NONE', *, *, #53550, .T. ) ;
#9224=CARTESIAN_POINT ( 'NONE',  ( -56.38001980572109062, 4.410024460692103077, 2.999999999999993339 ) ) ;
#9261=EDGE_LOOP ( 'NONE', ( #17584, #13863, #22718 ) ) ;
#9293=CARTESIAN_POINT ( 'NONE',  ( -37.09365488523594223, 9.510193405093987806, -4.936228699513737439 ) ) ;
#9299=CARTESIAN_POINT ( 'NONE',  ( -22.15441416008502529, 19.68629195356385964, 4.426028523006688253 ) ) ;
#9355=DIRECTION ( 'NONE',  ( 0.000000000000000000, 0.000000000000000000, 1.000000000000000000 ) ) ;
#9368=LINE ( 'NONE', #1409, #1533 ) ;
#9390=EDGE_LOOP ( 'NONE', ( #55400, #29866, #42316, #11635 ) ) ;
#9421=AXIS2_PLACEMENT_3D ( 'NONE', #23266, #27812, #32602 ) ;
#9426=DIRECTION ( 'NONE',  ( -0.7886751345948130876, 0.2113248654051844977, 0.5773502691896263972 ) ) ;
#9440=AXIS2_PLACEMENT_3D ( 'NONE', #51668, #7677, #38323 ) ;
#9510=CARTESIAN_POINT ( 'NONE',  ( -50.27554558092695913, 4.209026340267034705, 5.000000000000000000 ) ) ;
#9540=CARTESIAN_POINT ( 'NONE',  ( -15.35417357620467449, 23.79353959847493272, -3.874970200383425656 ) ) ;
#9565=B_SPLINE_CURVE_WITH_KNOTS ( 'NONE', 3,
 ( #16217, #12537, #21326, #12238 ),
 .UNSPECIFIED., .F., .F.,
 ( 4, 4 ),
 ( 0.000000000000000000, 0.0001352353904500101485 ),
 .UNSPECIFIED. ) ;
#9597=CARTESIAN_POINT ( 'NONE',  ( -50.45472955569960760, 3.742236127018431890, 5.000000000000000000 ) ) ;
#9600=CARTESIAN_POINT ( 'NONE',  ( -37.11431328563478615, 9.498266272062682702, -4.936536869034685360 ) ) ;
#9661=VECTOR ( 'NONE', #55067, 1000.000000000000114 ) ;
#9665=CARTESIAN_POINT ( 'NONE',  ( -20.63663879154963965, 20.74370688441071664, 4.329123301634322907 ) ) ;
#9673=CARTESIAN_POINT ( 'NONE',  ( -60.88973930853472183, 7.404220597074748333, 2.999999999999993339 ) ) ;
#9690=VERTEX_POINT ( 'NONE', #10975 ) ;
#9719=CARTESIAN_POINT ( 'NONE',  ( -24.57312748012714820, 18.34675972927921350, -4.549864808573585329 ) ) ;
#9741=DIRECTION ( 'NONE',  ( -1.000000000000000000, 0.000000000000000000, 0.000000000000000000 ) ) ;
#9747=ORIENTED_EDGE ( 'NONE', *, *, #32751, .T. ) ;
#9770=ORIENTED_EDGE ( 'NONE', *, *, #25414, .F. ) ;
#9773=EDGE_CURVE ( 'NONE', #31783, #27675, #1636, .T. ) ;
#9781=B_SPLINE_CURVE_WITH_KNOTS ( 'NONE', 3,
 ( #47430, #30413, #30699, #13628 ),
 .UNSPECIFIED., .F., .F.,
 ( 4, 4 ),
 ( 0.0001144323540671334324, 0.0003537324766284092063 ),
 .UNSPECIFIED. ) ;
#9795=CARTESIAN_POINT ( 'NONE',  ( -23.44701637808619665, 18.93456746265863799, 4.495868649597294819 ) ) ;
#9812=ORIENTED_EDGE ( 'NONE', *, *, #5926, .F. ) ;
#9859=EDGE_CURVE ( 'NONE', #32191, #49975, #53954, .T. ) ;
#9860=DIRECTION ( 'NONE',  ( 0.3535533905932738974, -0.6123724356957929160, 0.7071067811865487940 ) ) ;
#9868=CARTESIAN_POINT ( 'NONE',  ( -23.23471500290295921, 19.24370688441070953, 4.480778704491060971 ) ) ;
#9879=CARTESIAN_POINT ( 'NONE',  ( -38.32071399784587840, 8.801750496117048073, -4.953405659155169616 ) ) ;
#9915=FACE_OUTER_BOUND ( 'NONE', #51533, .T. ) ;
#9917=VERTEX_POINT ( 'NONE', #26555 ) ;
#9963=ORIENTED_EDGE ( 'NONE', *, *, #8674, .F. ) ;
#10058=EDGE_LOOP ( 'NONE', ( #48399, #39670, #10894, #44445 ) ) ;
#10085=CARTESIAN_POINT ( 'NONE',  ( -16.11986972353830083, 23.35146472169441267, -3.958709963775913554 ) ) ;
#10106=EDGE_LOOP ( 'NONE', ( #40506, #9747, #37023, #14379, #39036, #25268, #20038, #29547 ) ) ;
#10186=CARTESIAN_POINT ( 'NONE',  ( -25.54041736840764187, 17.91250900301538351, 4.591768117563441720 ) ) ;
#10197=CARTESIAN_POINT ( 'NONE',  ( -56.02165185617580079, 5.343604887189308705, 2.999999999999993339 ) ) ;
#10205=ORIENTED_EDGE ( 'NONE', *, *, #727, .F. ) ;
#10288=ORIENTED_EDGE ( 'NONE', *, *, #28680, .T. ) ;
#10303=ADVANCED_FACE ( 'NONE', ( #45833 ), #24268, .F. ) ;
#10308=EDGE_CURVE ( 'NONE', #48202, #45033, #46372, .T. ) ;
#10314=DIRECTION ( 'NONE',  ( 1.000000000000000000, 0.000000000000000000, -0.000000000000000000 ) ) ;
#10335=CARTESIAN_POINT ( 'NONE',  ( -21.64220182007004212, 20.16314479920728431, 4.391939828907996279 ) ) ;
#10356=CARTESIAN_POINT ( 'NONE',  ( -26.26580391614848864, 17.49370688441070953, -4.622528711259356271 ) ) ;
#10397=ORIENTED_EDGE ( 'NONE', *, *, #15013, .T. ) ;
#10399=LINE ( 'NONE', #1599, #34752 ) ;
#10403=VERTEX_POINT ( 'NONE', #25958 ) ;
#10460=EDGE_LOOP ( 'NONE', ( #20475, #13328, #28049 ) ) ;
#10469=EDGE_CURVE ( 'NONE', #44458, #50858, #1741, .T. ) ;
#10569=DIRECTION ( 'NONE',  ( -0.000000000000000000, -0.000000000000000000, -1.000000000000000000 ) ) ;
#10584=CARTESIAN_POINT ( 'NONE',  ( -24.96676581047183063, 18.24370688441070953, -4.657437592157546824 ) ) ;
#10614=ADVANCED_FACE ( 'NONE', ( #17015 ), #55074, .F. ) ;
#10653=VECTOR ( 'NONE', #42681, 1000.000000000000000 ) ;
#10668=ORIENTED_EDGE ( 'NONE', *, *, #44636, .F. ) ;
#10688=VERTEX_POINT ( 'NONE', #35729 ) ;
#10696=CARTESIAN_POINT ( 'NONE',  ( -19.33759994122731385, 21.49370731433205250, -4.239680377485293583 ) ) ;
#10706=EDGE_LOOP ( 'NONE', ( #45349, #39990, #19819, #15141 ) ) ;
#10723=CARTESIAN_POINT ( 'NONE',  ( -24.83619454210204580, 18.20872041849631984, -4.561852789702152577 ) ) ;
#10829=EDGE_CURVE ( 'NONE', #54076, #45033, #21954, .T. ) ;
#10849=CARTESIAN_POINT ( 'NONE',  ( -24.53374897521541698, 18.49370927080960669, -4.545578601930409413 ) ) ;
#10894=ORIENTED_EDGE ( 'NONE', *, *, #18197, .F. ) ;
#10936=CARTESIAN_POINT ( 'NONE',  ( -29.00661482377690703, 15.91129896909354180, 4.725528206980505352 ) ) ;
#10938=ORIENTED_EDGE ( 'NONE', *, *, #23443, .T. ) ;
#10948=CARTESIAN_POINT ( 'NONE',  ( -63.00984630926863161, 1.788483511016180305, 2.999999999999993339 ) ) ;
#10957=CARTESIAN_POINT ( 'NONE',  ( -29.02628690221330388, 15.89994128931277295, -4.726187803958536549 ) ) ;
#10967=CARTESIAN_POINT ( 'NONE',  ( -24.87971818958798309, 18.22038254469182661, -4.563127009718482618 ) ) ;
#10975=CARTESIAN_POINT ( 'NONE',  ( -27.13299098042555002, 16.99303619941258603, -4.657414165320978405 ) ) ;
#10981=CARTESIAN_POINT ( 'NONE',  ( -27.56460882755735753, 16.74384151918395247, 4.673983433494172779 ) ) ;
#11013=FACE_OUTER_BOUND ( 'NONE', #20075, .T. ) ;
#11046=VECTOR ( 'NONE', #18242, 1000.000000000000000 ) ;
#11088=DIRECTION ( 'NONE',  ( 0.3583679495452941066, 0.9335804264972041855, 0.000000000000000000 ) ) ;
#11092=CARTESIAN_POINT ( 'NONE',  ( -23.44701637808619665, 18.93456746265863799, 4.495868649597294819 ) ) ;
#11093=EDGE_CURVE ( 'NONE', #12998, #21622, #26288, .T. ) ;
#11134=CARTESIAN_POINT ( 'NONE',  ( -19.54294029912376729, 21.18270206417094315, -4.260498045023555669 ) ) ;
#11138=ORIENTED_EDGE ( 'NONE', *, *, #41766, .F. ) ;
#11163=EDGE_CURVE ( 'NONE', #34812, #49013, #3035, .T. ) ;
#11184=VECTOR ( 'NONE', #36642, 1000.000000000000000 ) ;
#11238=CARTESIAN_POINT ( 'NONE',  ( -37.63793934321780199, 10.92800143433129456, -4.933120776947167663 ) ) ;
#11260=CIRCLE ( 'NONE', #9440, 0.5000000000000004441 ) ;
#11295=ORIENTED_EDGE ( 'NONE', *, *, #10308, .T. ) ;
#11304=CARTESIAN_POINT ( 'NONE',  ( -11.36804826722768702, 24.91136206679766829, 3.000000000000000000 ) ) ;
#11317=CARTESIAN_POINT ( 'NONE',  ( -24.53375310857961367, 18.49370688441070953, 4.545578210335888159 ) ) ;
#11325=LINE ( 'NONE', #15311, #15717 ) ;
#11377=DIRECTION ( 'NONE',  ( 0.5000000000000011102, -0.8660254037844380415, 0.000000000000000000 ) ) ;
#11382=AXIS2_PLACEMENT_3D ( 'NONE', #6085, #23389, #40705 ) ;
#11412=LINE ( 'NONE', #3450, #17540 ) ;
#11435=ADVANCED_FACE ( 'NONE', ( #52613 ), #4382, .F. ) ;
#11479=ADVANCED_FACE ( 'NONE', ( #369 ), #43812, .F. ) ;
#11529=FACE_OUTER_BOUND ( 'NONE', #4360, .T. ) ;
#11537=CARTESIAN_POINT ( 'NONE',  ( -29.06878564040112067, 15.87540463137980851, -4.727619564647471684 ) ) ;
#11552=VERTEX_POINT ( 'NONE', #23086 ) ;
#11566=CARTESIAN_POINT ( 'NONE',  ( -21.93567689722629765, 19.99370688441071309, 4.408989160011352659 ) ) ;
#11568=EDGE_CURVE ( 'NONE', #2911, #38353, #22537, .T. ) ;
#11612=VERTEX_POINT ( 'NONE', #17905 ) ;
#11635=ORIENTED_EDGE ( 'NONE', *, *, #50425, .T. ) ;
#11660=PLANE ( 'NONE',  #24024 ) ;
#11712=LINE ( 'NONE', #15673, #32230 ) ;
#11745=ADVANCED_FACE ( 'NONE', ( #44549 ), #14471, .F. ) ;
#11752=DIRECTION ( 'NONE',  ( 0.8660254037844380415, 0.5000000000000011102, 0.000000000000000000 ) ) ;
#11762=CARTESIAN_POINT ( 'NONE',  ( -46.55906441860520317, 5.863990010960497656, -5.000000000000000000 ) ) ;
#11786=CARTESIAN_POINT ( 'NONE',  ( -26.03813301551774728, 17.43270265044663603, 4.490773887887535842 ) ) ;
#11819=B_SPLINE_CURVE_WITH_KNOTS ( 'NONE', 3,
 ( #4701, #34519, #43346, #3851 ),
 .UNSPECIFIED., .F., .F.,
 ( 4, 4 ),
 ( 0.0002388585478777321643, 0.0002669665482816597568 ),
 .UNSPECIFIED. ) ;
#11908=CARTESIAN_POINT ( 'NONE',  ( -26.25138199253913385, 17.50203338588876179, 4.621929860192643069 ) ) ;
#11965=LINE ( 'NONE', #50870, #22209 ) ;
#11988=DIRECTION ( 'NONE',  ( 1.007958083594381472E-15, -3.869188571150965146E-16, 1.000000000000000000 ) ) ;
#12018=DIRECTION ( 'NONE',  ( 0.2113248654051873565, 0.7886751345948123104, 0.5773502691896265082 ) ) ;
#12055=CARTESIAN_POINT ( 'NONE',  ( -19.65677579747983472, 21.21320419402555402, 4.265613255886147925 ) ) ;
#12058=DIRECTION ( 'NONE',  ( 0.5000000000000011102, -0.8660254037844380415, 0.000000000000000000 ) ) ;
#12156=FACE_OUTER_BOUND ( 'NONE', #39852, .T. ) ;
#12160=LINE ( 'NONE', #29495, #53719 ) ;
#12161=CARTESIAN_POINT ( 'NONE',  ( -19.66742376178725493, 19.57123263517775769, 4.314754536491465231 ) ) ;
#12172=CARTESIAN_POINT ( 'NONE',  ( -50.27554558092695913, 4.209026340267034705, 5.000000000000000000 ) ) ;
#12188=LINE ( 'NONE', #47110, #616 ) ;
#12220=CARTESIAN_POINT ( 'NONE',  ( -46.27156441860557123, 5.366025403784241199, -5.000000000000000000 ) ) ;
#12232=CARTESIAN_POINT ( 'NONE',  ( -22.04728230093569152, 19.65758605842115969, -4.422151119964278010 ) ) ;
#12238=CARTESIAN_POINT ( 'NONE',  ( -24.83619032682412353, 18.20871928901600256, 4.561852666301203563 ) ) ;
#12263=AXIS2_PLACEMENT_3D ( 'NONE', #9082, #9355, #36071 ) ;
#12289=AXIS2_PLACEMENT_3D ( 'NONE', #17929, #22472, #44029 ) ;
#12341=EDGE_CURVE ( 'NONE', #34812, #24159, #18096, .T. ) ;
#12348=CARTESIAN_POINT ( 'NONE',  ( -11.64304826722768382, 25.38767603887911051, -3.000000000000000000 ) ) ;
#12363=CARTESIAN_POINT ( 'NONE',  ( -12.29957260759845106, 23.82506348239776273, -3.515194272803603415 ) ) ;
#12384=VECTOR ( 'NONE', #6896, 1000.000000000000000 ) ;
#12436=ORIENTED_EDGE ( 'NONE', *, *, #15634, .F. ) ;
#12442=DIRECTION ( 'NONE',  ( 0.3535533905932752297, -0.6123724356957952475, -0.7071067811865462405 ) ) ;
#12491=ORIENTED_EDGE ( 'NONE', *, *, #19403, .F. ) ;
#12515=EDGE_CURVE ( 'NONE', #42394, #52748, #6263, .T. ) ;
#12516=B_SPLINE_CURVE_WITH_KNOTS ( 'NONE', 3,
 ( #44984, #31363, #697, #9795 ),
 .UNSPECIFIED., .F., .F.,
 ( 4, 4 ),
 ( 0.0001724778598249929792, 0.0003421153678589267371 ),
 .UNSPECIFIED. ) ;
#12537=CARTESIAN_POINT ( 'NONE',  ( -24.92324054119748311, 18.23204432365830030, 4.564397195367118520 ) ) ;
#12546=DIRECTION ( 'NONE',  ( 0.9659258262890682012, -0.2588190451025213501, 0.000000000000000000 ) ) ;
#12577=FACE_OUTER_BOUND ( 'NONE', #50426, .T. ) ;
#12661=CARTESIAN_POINT ( 'NONE',  ( -22.94167088982010583, 19.41289598198349253, 4.465499946586994895 ) ) ;
#12681=VERTEX_POINT ( 'NONE', #8969 ) ;
#12684=VERTEX_POINT ( 'NONE', #9224 ) ;
#12753=FACE_OUTER_BOUND ( 'NONE', #23953, .T. ) ;
#12794=LINE ( 'NONE', #30117, #15507 ) ;
#12836=EDGE_CURVE ( 'NONE', #25142, #26953, #35635, .T. ) ;
#12965=EDGE_LOOP ( 'NONE', ( #22878, #54116, #33746, #54474, #19413, #6689 ) ) ;
#12987=EDGE_CURVE ( 'NONE', #29855, #15218, #50367, .T. ) ;
#12998=VERTEX_POINT ( 'NONE', #54342 ) ;
#13017=DIRECTION ( 'NONE',  ( -1.000000000000000000, 0.000000000000000000, 0.000000000000000000 ) ) ;
#13099=EDGE_CURVE ( 'NONE', #44683, #48518, #9368, .T. ) ;
#13160=CLOSED_SHELL ( 'NONE', ( #43827, #29227, #10303, #44606, #53124, #11479, #44827, #54797, #35461, #17663, #28041, #14786, #3976, #6857, #17209, #55333, #11745, #53873, #10614, #49999, #27367, #4945, #44545, #11435, #47399, #6321, #54230, #41877, #33767, #22103, #3275, #22660, #54366, #49968, #45435, #15902, #44436, #51617, #34084, #56080, #5233, #36232, #18692, #53536, #533, #22020, #21448, #26237, #52711, #21500, #27690, #14677, #18516, #18199, #50674 ) ) ;
#13193=EDGE_LOOP ( 'NONE', ( #52620, #48064, #37638, #53051 ) ) ;
#13220=DIRECTION ( 'NONE',  ( 0.000000000000000000, 0.000000000000000000, 1.000000000000000000 ) ) ;
#13242=CARTESIAN_POINT ( 'NONE',  ( -46.02156441860523017, 4.933012701892206309, 5.000000000000000000 ) ) ;
#13280=DIRECTION ( 'NONE',  ( 0.3535533905932738974, -0.6123724356957929160, 0.7071067811865487940 ) ) ;
#13287=AXIS2_PLACEMENT_3D ( 'NONE', #22467, #31244, #14764 ) ;
#13288=CARTESIAN_POINT ( 'NONE',  ( -50.27554558092695913, 4.209026340267034705, 5.000000000000000000 ) ) ;
#13302=AXIS2_PLACEMENT_3D ( 'NONE', #12172, #16160, #20707 ) ;
#13304=CARTESIAN_POINT ( 'NONE',  ( -37.69457521496538277, 9.163251890963174162, -4.944930165255981613 ) ) ;
#13307=DIRECTION ( 'NONE',  ( -0.8660254037844379305, -0.5000000000000011102, 0.000000000000000000 ) ) ;
#13310=ORIENTED_EDGE ( 'NONE', *, *, #51462, .T. ) ;
#13328=ORIENTED_EDGE ( 'NONE', *, *, #33811, .T. ) ;
#13366=CARTESIAN_POINT ( 'NONE',  ( -50.45472955569960760, 3.742236127018431890, 5.000000000000000000 ) ) ;
#13373=DIRECTION ( 'NONE',  ( 0.000000000000000000, 0.000000000000000000, 1.000000000000000000 ) ) ;
#13390=APPLICATION_CONTEXT ( 'automotive_design' ) ;
#13433=DIRECTION ( 'NONE',  ( 0.5000000000000011102, -0.8660254037844380415, 0.000000000000000000 ) ) ;
#13452=CARTESIAN_POINT ( 'NONE',  ( -11.38054826722768276, 24.93301270189227736, -3.000000000000000000 ) ) ;
#13492=EDGE_CURVE ( 'NONE', #7274, #30542, #40027, .T. ) ;
#13505=CARTESIAN_POINT ( 'NONE',  ( -61.10213307005877681, 6.758246409053505488, -3.000000000000007105 ) ) ;
#13515=CARTESIAN_POINT ( 'NONE',  ( -13.57018763683711349, 24.82352436079930769, -3.618365315326378173 ) ) ;
#13517=B_SPLINE_CURVE_WITH_KNOTS ( 'NONE', 3,
 ( #36701, #6887, #49490, #6589 ),
 .UNSPECIFIED., .F., .F.,
 ( 4, 4 ),
 ( 0.000000000000000000, 0.0003539001916872983413 ),
 .UNSPECIFIED. ) ;
#13565=CARTESIAN_POINT ( 'NONE',  ( -19.68185725454445034, 19.56289945424903109, -4.315709269779091528 ) ) ;
#13574=PRODUCT_DEFINITION_FORMATION_WITH_SPECIFIED_SOURCE ( 'ANY', '', #31892, .NOT_KNOWN. ) ;
#13575=DIRECTION ( 'NONE',  ( 0.000000000000000000, 0.000000000000000000, 1.000000000000000000 ) ) ;
#13607=CARTESIAN_POINT ( 'NONE',  ( -25.25174164940481347, 18.07917600709017947, 4.578957096563475382 ) ) ;
#13626=B_SPLINE_CURVE_WITH_KNOTS ( 'NONE', 3,
 ( #5307, #22618, #14105, #10696 ),
 .UNSPECIFIED., .F., .F.,
 ( 4, 4 ),
 ( 0.000000000000000000, 0.0003539001916874550085 ),
 .UNSPECIFIED. ) ;
#13628=CARTESIAN_POINT ( 'NONE',  ( -23.23471098716119698, 19.24370920290025566, -4.480780584866845828 ) ) ;
#13696=AXIS2_PLACEMENT_3D ( 'NONE', #41721, #54499, #2812 ) ;
#13717=EDGE_CURVE ( 'NONE', #43487, #24159, #54742, .T. ) ;
#13725=ORIENTED_EDGE ( 'NONE', *, *, #39119, .T. ) ;
#13778=LINE ( 'NONE', #22328, #52275 ) ;
#13833=CARTESIAN_POINT ( 'NONE',  ( -15.40229489717257394, 22.03370593329148264, -3.962133388944282686 ) ) ;
#13857=ORIENTED_EDGE ( 'NONE', *, *, #44373, .F. ) ;
#13863=ORIENTED_EDGE ( 'NONE', *, *, #33593, .T. ) ;
#13937=ORIENTED_EDGE ( 'NONE', *, *, #34493, .F. ) ;
#13942=LINE ( 'NONE', #48876, #32736 ) ;
#13968=CARTESIAN_POINT ( 'NONE',  ( -22.02718324817240969, 19.65220053346460460, 4.407440554554201917 ) ) ;
#13980=EDGE_CURVE ( 'NONE', #24541, #2142, #55450, .T. ) ;
#14093=VERTEX_POINT ( 'NONE', #16283 ) ;
#14105=CARTESIAN_POINT ( 'NONE',  ( -19.36810218178845489, 21.37987375194732209, -4.244941833920536922 ) ) ;
#14115=VECTOR ( 'NONE', #54871, 1000.000000000000000 ) ;
#14140=CARTESIAN_POINT ( 'NONE',  ( -20.22851404498383587, 19.24728700913452073, -4.351128180092163511 ) ) ;
#14147=B_SPLINE_CURVE_WITH_KNOTS ( 'NONE', 3,
 ( #8982, #13242, #18311, #22023 ),
 .UNSPECIFIED., .F., .F.,
 ( 4, 4 ),
 ( 0.000000000000000000, 1.000000000000000000 ),
 .UNSPECIFIED. ) ;
#14199=DIRECTION ( 'NONE',  ( 0.9659258262890692004, -0.2588190451025176864, 0.000000000000000000 ) ) ;
#14203=B_SPLINE_CURVE_WITH_KNOTS ( 'NONE', 3,
 ( #27946, #44982, #49520, #27097 ),
 .UNSPECIFIED., .F., .F.,
 ( 4, 4 ),
 ( 0.7664662348551912752, 1.000000000000000000 ),
 .UNSPECIFIED. ) ;
#14220=SURFACE_SIDE_STYLE ('',( #31532 ) ) ;
#14284=DIRECTION ( 'NONE',  ( -0.2588190451025176864, -0.9659258262890692004, 0.000000000000000000 ) ) ;
#14291=EDGE_CURVE ( 'NONE', #46324, #40047, #20253, .T. ) ;
#14347=CARTESIAN_POINT ( 'NONE',  ( -22.36868959911851462, 19.74370688441071309, -4.657437592157546824 ) ) ;
#14369=CARTESIAN_POINT ( 'NONE',  ( -13.93117922710646539, 24.61510576898210445, -3.677906343404563572 ) ) ;
#14379=ORIENTED_EDGE ( 'NONE', *, *, #30791, .F. ) ;
#14385=CARTESIAN_POINT ( 'NONE',  ( -27.99202758151029613, 16.49707118653253346, 4.690121163682637651 ) ) ;
#14395=ORIENTED_EDGE ( 'NONE', *, *, #55203, .F. ) ;
#14428=CARTESIAN_POINT ( 'NONE',  ( -28.19207438693690904, 14.64952330200006259, 4.723338118696758237 ) ) ;
#14471=PLANE ( 'NONE',  #38622 ) ;
#14475=DIRECTION ( 'NONE',  ( -0.5000000000000015543, 0.8660254037844378194, 0.000000000000000000 ) ) ;
#14517=CARTESIAN_POINT ( 'NONE',  ( -50.45472955569960760, 3.742236127018431890, -5.000000000000000000 ) ) ;
#14520=CARTESIAN_POINT ( 'NONE',  ( -61.70068505767310540, 8.059153983834628221, -5.000000000000000000 ) ) ;
#14552=EDGE_CURVE ( 'NONE', #53976, #19985, #24884, .T. ) ;
#14561=CARTESIAN_POINT ( 'NONE',  ( -61.21055533376208047, 7.871010810323351592, 5.000000000000012434 ) ) ;
#14635=VECTOR ( 'NONE', #13575, 1000.000000000000000 ) ;
#14656=CARTESIAN_POINT ( 'NONE',  ( -46.52156441860571334, 5.799038105676371124, -5.000000000000000000 ) ) ;
#14677=ADVANCED_FACE ( 'NONE', ( #29856 ), #39502, .T. ) ;
#14764=DIRECTION ( 'NONE',  ( -0.3583679495452925523, -0.9335804264972047406, 0.000000000000000000 ) ) ;
#14786=ADVANCED_FACE ( 'NONE', ( #1123 ), #40326, .T. ) ;
#14862=LINE ( 'NONE', #27940, #14993 ) ;
#14884=CARTESIAN_POINT ( 'NONE',  ( -45.77156441860525149, 4.499999999999981348, -5.000000000000000000 ) ) ;
#14921=VECTOR ( 'NONE', #9021, 1000.000000000000000 ) ;
#14925=VECTOR ( 'NONE', #34268, 1000.000000000000114 ) ;
#14984=CARTESIAN_POINT ( 'NONE',  ( -23.27598484286411562, 19.08968574485540515, 4.485782763162093900 ) ) ;
#14993=VECTOR ( 'NONE', #29029, 1000.000000000000114 ) ;
#15013=EDGE_CURVE ( 'NONE', #37067, #39800, #42753, .T. ) ;
#15020=CARTESIAN_POINT ( 'NONE',  ( -11.36804826722768347, 24.91136206679770382, 5.000000000000000888 ) ) ;
#15033=CARTESIAN_POINT ( 'NONE',  ( -50.02554558092695913, 3.776013638374817294, 5.000000000000000000 ) ) ;
#15072=CARTESIAN_POINT ( 'NONE',  ( -50.99228148001754590, 2.341865487272627000, 5.000000000000000000 ) ) ;
#15079=VECTOR ( 'NONE', #35338, 1000.000000000000000 ) ;
#15082=EDGE_CURVE ( 'NONE', #24541, #7274, #13778, .T. ) ;
#15132=B_SPLINE_CURVE_WITH_KNOTS ( 'NONE', 3,
 ( #31658, #28208, #32212, #19707 ),
 .UNSPECIFIED., .F., .F.,
 ( 4, 4 ),
 ( 0.000000000000000000, 0.0001521986025861482247 ),
 .UNSPECIFIED. ) ;
#15141=ORIENTED_EDGE ( 'NONE', *, *, #11568, .T. ) ;
#15174=VERTEX_POINT ( 'NONE', #41016 ) ;
#15186=CARTESIAN_POINT ( 'NONE',  ( -26.84049344369173085, 17.16190973098311900, -4.646098577050644884 ) ) ;
#15218=VERTEX_POINT ( 'NONE', #32245 ) ;
#15220=ORIENTED_EDGE ( 'NONE', *, *, #55262, .T. ) ;
#15234=FACE_OUTER_BOUND ( 'NONE', #4852, .T. ) ;
#15242=CARTESIAN_POINT ( 'NONE',  ( -29.11308221448052080, 15.84982999241088919, -4.729108557267000634 ) ) ;
#15256=CARTESIAN_POINT ( 'NONE',  ( -50.99228148001754590, 2.341865487272625668, 2.999999999999993339 ) ) ;
#15295=CARTESIAN_POINT ( 'NONE',  ( -24.57312748012714820, 18.34675972927921350, -4.549864808573585329 ) ) ;
#15311=CARTESIAN_POINT ( 'NONE',  ( -64.10539783498545319, 7.375519243179410545, -3.000000000000000000 ) ) ;
#15341=FACE_OUTER_BOUND ( 'NONE', #10058, .T. ) ;
#15371=DIRECTION ( 'NONE',  ( 0.5000000000000011102, -0.8660254037844380415, 0.000000000000000000 ) ) ;
#15393=ORIENTED_EDGE ( 'NONE', *, *, #52441, .F. ) ;
#15471=CARTESIAN_POINT ( 'NONE',  ( -26.25138199253913385, 17.50203338588876179, 4.621929860192643069 ) ) ;
#15478=LINE ( 'NONE', #19759, #26888 ) ;
#15498=CARTESIAN_POINT ( 'NONE',  ( -24.53374897521541698, 18.49370927080960669, -4.545578601930409413 ) ) ;
#15507=VECTOR ( 'NONE', #43204, 1000.000000000000000 ) ;
#15547=CARTESIAN_POINT ( 'NONE',  ( -45.73406441860519323, 4.435048094716154132, 5.000000000000000000 ) ) ;
#15589=CIRCLE ( 'NONE', #16527, 0.5000000000000004441 ) ;
#15617=CARTESIAN_POINT ( 'NONE',  ( -50.27554558092695913, 4.209026340267034705, -5.000000000000000000 ) ) ;
#15634=EDGE_CURVE ( 'NONE', #34711, #3752, #35646, .T. ) ;
#15673=CARTESIAN_POINT ( 'NONE',  ( -26.26580391614848864, 17.49370688441070953, -4.657437592157546824 ) ) ;
#15703=EDGE_LOOP ( 'NONE', ( #32125, #29376, #46729, #17872 ) ) ;
#15717=VECTOR ( 'NONE', #16150, 1000.000000000000000 ) ;
#15813=LINE ( 'NONE', #54426, #21461 ) ;
#15824=VECTOR ( 'NONE', #49891, 1000.000000000000000 ) ;
#15846=PLANE ( 'NONE',  #20155 ) ;
#15854=CARTESIAN_POINT ( 'NONE',  ( -50.02554558092695913, 3.776013638374815962, -5.000000000000000000 ) ) ;
#15888=AXIS2_PLACEMENT_3D ( 'NONE', #49164, #53177, #9741 ) ;
#15902=ADVANCED_FACE ( 'NONE', ( #47180 ), #42641, .F. ) ;
#15955=ORIENTED_EDGE ( 'NONE', *, *, #20596, .T. ) ;
#15988=EDGE_LOOP ( 'NONE', ( #42781, #28738, #34162 ) ) ;
#16005=DIRECTION ( 'NONE',  ( 0.2113248654051873565, 0.7886751345948121994, -0.5773502691896263972 ) ) ;
#16027=ORIENTED_EDGE ( 'NONE', *, *, #13717, .T. ) ;
#16031=LINE ( 'NONE', #33606, #10653 ) ;
#16040=ORIENTED_EDGE ( 'NONE', *, *, #27250, .T. ) ;
#16055=CIRCLE ( 'NONE', #8818, 2.000000000000001776 ) ;
#16089=LINE ( 'NONE', #15256, #5809 ) ;
#16114=VERTEX_POINT ( 'NONE', #32940 ) ;
#16150=DIRECTION ( 'NONE',  ( -0.3583679495452925523, -0.9335804264972047406, -0.000000000000000000 ) ) ;
#16160=DIRECTION ( 'NONE',  ( -0.000000000000000000, 0.000000000000000000, -1.000000000000000000 ) ) ;
#16217=CARTESIAN_POINT ( 'NONE',  ( -24.96676581047183063, 18.24370688441070953, 4.565775410814726598 ) ) ;
#16221=LINE ( 'NONE', #25312, #28429 ) ;
#16245=DIRECTION ( 'NONE',  ( 0.9659258262890692004, -0.2588190451025176864, 0.000000000000000000 ) ) ;
#16261=CARTESIAN_POINT ( 'NONE',  ( -62.23823698199102950, 6.658783344088819334, 5.000000000000000000 ) ) ;
#16275=DIRECTION ( 'NONE',  ( 0.000000000000000000, 0.000000000000000000, 1.000000000000000000 ) ) ;
#16283=CARTESIAN_POINT ( 'NONE',  ( -22.02718324817240969, 19.65220053346460816, -4.407437592157546824 ) ) ;
#16361=EDGE_CURVE ( 'NONE', #39727, #42260, #1307, .T. ) ;
#16386=FACE_OUTER_BOUND ( 'NONE', #41236, .T. ) ;
#16394=CARTESIAN_POINT ( 'NONE',  ( -25.83279121425626812, 17.74370688441070953, 4.657440554554202805 ) ) ;
#16395=ORIENTED_EDGE ( 'NONE', *, *, #26676, .T. ) ;
#16410=CARTESIAN_POINT ( 'NONE',  ( -11.13274803382162226, 24.49872996416489457, 3.250237613767693823 ) ) ;
#16490=CARTESIAN_POINT ( 'NONE',  ( -25.84533184003709039, 17.69690463183794193, -4.605409455127198015 ) ) ;
#16501=ORIENTED_EDGE ( 'NONE', *, *, #45209, .T. ) ;
#16527=AXIS2_PLACEMENT_3D ( 'NONE', #15617, #42026, #23871 ) ;
#16551=CARTESIAN_POINT ( 'NONE',  ( -23.34675887425330743, 18.98665486385284495, -4.490845947935475202 ) ) ;
#16580=VERTEX_POINT ( 'NONE', #21981 ) ;
#16586=ORIENTED_EDGE ( 'NONE', *, *, #36974, .T. ) ;
#16647=CARTESIAN_POINT ( 'NONE',  ( -60.74376512051347987, 7.691826835550698682, -3.000000000000007105 ) ) ;
#16654=ORIENTED_EDGE ( 'NONE', *, *, #15634, .T. ) ;
#16685=B_SPLINE_CURVE_WITH_KNOTS ( 'NONE', 3,
 ( #12232, #43714, #56230, #47993 ),
 .UNSPECIFIED., .F., .F.,
 ( 4, 4 ),
 ( 2.082079450497559408E-05, 0.0003537660668259436916 ),
 .UNSPECIFIED. ) ;
#16707=CARTESIAN_POINT ( 'NONE',  ( -26.95299377262630003, 15.36490682821995257, 4.679584696907975960 ) ) ;
#16723=EDGE_CURVE ( 'NONE', #45033, #16580, #12516, .T. ) ;
#16749=EDGE_CURVE ( 'NONE', #19901, #37705, #43839, .T. ) ;
#16790=EDGE_CURVE ( 'NONE', #27945, #607, #40448, .T. ) ;
#16793=CARTESIAN_POINT ( 'NONE',  ( -21.93567689722629765, 19.99370688441071309, -4.657437592157546824 ) ) ;
#16839=CARTESIAN_POINT ( 'NONE',  ( -50.27554558092695913, 4.209026340267034705, -5.000000000000000000 ) ) ;
#16876=CARTESIAN_POINT ( 'NONE',  ( -24.73909490984108928, 18.18270265044663603, 4.490773887887535842 ) ) ;
#16909=DIRECTION ( 'NONE',  ( 0.8660254037844380415, 0.5000000000000011102, 0.000000000000000000 ) ) ;
#16971=ORIENTED_EDGE ( 'NONE', *, *, #13099, .T. ) ;
#16976=PLANE ( 'NONE',  #531 ) ;
#16981=VECTOR ( 'NONE', #1765, 1000.000000000000000 ) ;
#17003=CARTESIAN_POINT ( 'NONE',  ( -19.67298185230172436, 19.56802367012303989, 4.315122289059762473 ) ) ;
#17015=FACE_OUTER_BOUND ( 'NONE', #10106, .T. ) ;
#17024=VERTEX_POINT ( 'NONE', #34425 ) ;
#17093=DIRECTION ( 'NONE',  ( 0.3535533905932738974, -0.6123724356957929160, 0.7071067811865487940 ) ) ;
#17108=DIRECTION ( 'NONE',  ( -1.000000000000000000, 0.000000000000000000, 0.000000000000000000 ) ) ;
#17109=FACE_OUTER_BOUND ( 'NONE', #2683, .T. ) ;
#17122=DIRECTION ( 'NONE',  ( -0.3583679495452941066, -0.9335804264972041855, 0.000000000000000000 ) ) ;
#17159=CARTESIAN_POINT ( 'NONE',  ( -20.63663870328428374, 20.74370693537071020, -4.329125112780540796 ) ) ;
#17166=CARTESIAN_POINT ( 'NONE',  ( -11.13054826722768098, 24.50000000000005684, -3.000000000000000000 ) ) ;
#17209=ADVANCED_FACE ( 'NONE', ( #2568 ), #11660, .T. ) ;
#17293=EDGE_CURVE ( 'NONE', #10403, #36742, #19626, .T. ) ;
#17364=CARTESIAN_POINT ( 'NONE',  ( -56.20083583094844926, 4.876814673940706335, -3.000000000000007105 ) ) ;
#17427=CARTESIAN_POINT ( 'NONE',  ( -15.34211164085077783, 22.06845275252959127, -3.955769444135373014 ) ) ;
#17476=CARTESIAN_POINT ( 'NONE',  ( -11.88054826722767743, 25.79903810567671840, -3.133157401209314852 ) ) ;
#17479=ORIENTED_EDGE ( 'NONE', *, *, #33655, .F. ) ;
#17518=CARTESIAN_POINT ( 'NONE',  ( -23.23471098716119698, 19.24370920290025566, -4.480780584866845828 ) ) ;
#17540=VECTOR ( 'NONE', #33823, 1000.000000000000114 ) ;
#17541=CARTESIAN_POINT ( 'NONE',  ( -17.66651931516290475, 20.72645535605904499, -4.173277724953098122 ) ) ;
#17567=VERTEX_POINT ( 'NONE', #15295 ) ;
#17573=EDGE_CURVE ( 'NONE', #30957, #2911, #39434, .T. ) ;
#17583=DIRECTION ( 'NONE',  ( 0.000000000000000000, 0.000000000000000000, 1.000000000000000000 ) ) ;
#17584=ORIENTED_EDGE ( 'NONE', *, *, #30721, .F. ) ;
#17630=CARTESIAN_POINT ( 'NONE',  ( -19.33760068587298164, 21.49370688441072019, -4.657437592157546824 ) ) ;
#17656=CIRCLE ( 'NONE', #52107, 0.5000000000000004441 ) ;
#17663=ADVANCED_FACE ( 'NONE', ( #11013 ), #2800, .T. ) ;
#17723=CARTESIAN_POINT ( 'NONE',  ( -20.66714045964585722, 20.62987310936006224, -4.333808234692209105 ) ) ;
#17737=CARTESIAN_POINT ( 'NONE',  ( -26.26580391614848864, 17.49370688441070953, -4.657437592157546824 ) ) ;
#17743=CARTESIAN_POINT ( 'NONE',  ( -19.77061338776520216, 21.24370688441071664, 4.270755533188014930 ) ) ;
#17756=VECTOR ( 'NONE', #55423, 1000.000000000000000 ) ;
#17761=EDGE_LOOP ( 'NONE', ( #36576, #8990, #43974, #33579, #44151, #28766, #16586, #48595, #5862, #32120 ) ) ;
#17798=VECTOR ( 'NONE', #40859, 1000.000000000000000 ) ;
#17806=EDGE_LOOP ( 'NONE', ( #38176, #2686, #6580, #33348 ) ) ;
#17843=CARTESIAN_POINT ( 'NONE',  ( -21.95272886865376094, 18.25181111654794108, -4.454155209268523485 ) ) ;
#17872=ORIENTED_EDGE ( 'NONE', *, *, #44141, .T. ) ;
#17900=DIRECTION ( 'NONE',  ( -0.3583679495452941621, -0.9335804264972042965, 0.000000000000000000 ) ) ;
#17905=CARTESIAN_POINT ( 'NONE',  ( -61.74810725808001877, 6.470640170577544481, 2.999999999999993339 ) ) ;
#17926=B_SPLINE_CURVE_WITH_KNOTS ( 'NONE', 3,
 ( #10356, #53505, #15186, #5816 ),
 .UNSPECIFIED., .F., .F.,
 ( 4, 4 ),
 ( 0.4250098312019520708, 0.4483797419119410210 ),
 .UNSPECIFIED. ) ;
#17929=CARTESIAN_POINT ( 'NONE',  ( -50.27554558092695913, 4.209026340267034705, -5.000000000000000000 ) ) ;
#17998=AXIS2_PLACEMENT_3D ( 'NONE', #22988, #18747, #14475 ) ;
#17999=PLANE ( 'NONE',  #42076 ) ;
#18018=CARTESIAN_POINT ( 'NONE',  ( -19.42910703681909368, 21.15220053346460816, 4.255330291687501543 ) ) ;
#18038=FACE_OUTER_BOUND ( 'NONE', #43628, .T. ) ;
#18048=PRODUCT_DEFINITION ( 'UNKNOWN', '', #13574, #6432 ) ;
#18051=CARTESIAN_POINT ( 'NONE',  ( -19.33759994122731385, 21.49370731433205250, -4.239680377485293583 ) ) ;
#18091=CARTESIAN_POINT ( 'NONE',  ( -23.23471500290295921, 19.24370688441070953, 4.657440554554202805 ) ) ;
#18096=LINE ( 'NONE', #4487, #55937 ) ;
#18099=CARTESIAN_POINT ( 'NONE',  ( -15.60496230262594608, 21.91669585219702654, -3.983230142812006047 ) ) ;
#18112=LINE ( 'NONE', #41309, #22311 ) ;
#18177=PLANE ( 'NONE',  #12289 ) ;
#18197=EDGE_CURVE ( 'NONE', #19901, #51242, #48312, .T. ) ;
#18199=ADVANCED_FACE ( 'NONE', ( #9143 ), #23056, .T. ) ;
#18217=DIRECTION ( 'NONE',  ( 0.8660254037844380415, 0.5000000000000011102, 0.000000000000000000 ) ) ;
#18218=EDGE_CURVE ( 'NONE', #2911, #42260, #44918, .T. ) ;
#18232=CARTESIAN_POINT ( 'NONE',  ( -25.85160216376510434, 17.67350346510513148, -4.606045122360801436 ) ) ;
#18236=ORIENTED_EDGE ( 'NONE', *, *, #50895, .F. ) ;
#18242=DIRECTION ( 'NONE',  ( -0.000000000000000000, -0.000000000000000000, -1.000000000000000000 ) ) ;
#18278=FILL_AREA_STYLE ('',( #951 ) ) ;
#18291=PLANE ( 'NONE',  #46508 ) ;
#18292=CARTESIAN_POINT ( 'NONE',  ( -20.95581447963228783, 20.46320434849166858, 4.352198852484694847 ) ) ;
#18311=CARTESIAN_POINT ( 'NONE',  ( -46.27156441860520175, 5.366025403784440151, 5.000000000000000000 ) ) ;
#18361=PLANE ( 'NONE',  #35794 ) ;
#18397=VECTOR ( 'NONE', #43271, 1000.000000000000000 ) ;
#18494=ORIENTED_EDGE ( 'NONE', *, *, #55454, .F. ) ;
#18516=ADVANCED_FACE ( 'NONE', ( #26138 ), #43447, .T. ) ;
#18568=ORIENTED_EDGE ( 'NONE', *, *, #13099, .F. ) ;
#18575=SURFACE_SIDE_STYLE ('',( #35610 ) ) ;
#18580=CARTESIAN_POINT ( 'NONE',  ( -25.83278826518980154, 17.74370858705499288, -4.604226652742015702 ) ) ;
#18692=ADVANCED_FACE ( 'NONE', ( #30686 ), #44843, .F. ) ;
#18747=DIRECTION ( 'NONE',  ( 0.8660254037844378194, 0.5000000000000015543, -0.000000000000000000 ) ) ;
#18779=VERTEX_POINT ( 'NONE', #11317 ) ;
#18790=DIRECTION ( 'NONE',  ( -0.000000000000000000, -0.000000000000000000, 1.000000000000000000 ) ) ;
#18824=EDGE_CURVE ( 'NONE', #49013, #43487, #23544, .T. ) ;
#18866=DIRECTION ( 'NONE',  ( -0.000000000000000000, -0.000000000000000000, 1.000000000000000000 ) ) ;
#18917=ORIENTED_EDGE ( 'NONE', *, *, #18824, .F. ) ;
#18926=ORIENTED_EDGE ( 'NONE', *, *, #51462, .F. ) ;
#18960=EDGE_CURVE ( 'NONE', #3752, #18987, #54913, .T. ) ;
#18961=CARTESIAN_POINT ( 'NONE',  ( -28.28184430289702789, 14.59769461685536740, 4.726375084653139602 ) ) ;
#18963=CARTESIAN_POINT ( 'NONE',  ( -63.00984630926864583, 1.788483511016180305, -3.000000000000007105 ) ) ;
#18987=VERTEX_POINT ( 'NONE', #34760 ) ;
#19018=LINE ( 'NONE', #23297, #8821 ) ;
#19028=ORIENTED_EDGE ( 'NONE', *, *, #13980, .T. ) ;
#19037=ORIENTED_EDGE ( 'NONE', *, *, #42845, .F. ) ;
#19152=CARTESIAN_POINT ( 'NONE',  ( -20.42931928434034461, 20.86340285770621961, -4.315541546191446365 ) ) ;
#19156=CARTESIAN_POINT ( 'NONE',  ( -22.04727804374295275, 19.65758491770980143, 4.422150965879553475 ) ) ;
#19165=EDGE_CURVE ( 'NONE', #49975, #6581, #11712, .T. ) ;
#19168=CARTESIAN_POINT ( 'NONE',  ( -29.13153550921558121, 15.83917597772816244, 4.729727457563339676 ) ) ;
#19187=VERTEX_POINT ( 'NONE', #36725 ) ;
#19301=ORIENTED_EDGE ( 'NONE', *, *, #38882, .T. ) ;
#19303=LINE ( 'NONE', #41173, #11184 ) ;
#19313=CARTESIAN_POINT ( 'NONE',  ( -26.25138199253913385, 17.50203338588876179, 4.621929860192643069 ) ) ;
#19357=STYLED_ITEM ( 'NONE', ( #50343 ), #41257 ) ;
#19403=EDGE_CURVE ( 'NONE', #31783, #5918, #32274, .T. ) ;
#19413=ORIENTED_EDGE ( 'NONE', *, *, #10469, .T. ) ;
#19425=VECTOR ( 'NONE', #44216, 1000.000000000000000 ) ;
#19434=EDGE_CURVE ( 'NONE', #54860, #6825, #33854, .T. ) ;
#19472=CARTESIAN_POINT ( 'NONE',  ( -23.66772770479517618, 18.99370688441070953, -4.657437592157546824 ) ) ;
#19482=CARTESIAN_POINT ( 'NONE',  ( -30.26074760107038131, 15.18722507252361709, -4.766914839722605102 ) ) ;
#19531=ORIENTED_EDGE ( 'NONE', *, *, #21234, .T. ) ;
#19603=ORIENTED_EDGE ( 'NONE', *, *, #7154, .T. ) ;
#19626=LINE ( 'NONE', #1988, #28560 ) ;
#19637=CARTESIAN_POINT ( 'NONE',  ( -23.59415687586314547, 18.97399364021188717, 4.500635337789387513 ) ) ;
#19645=ORIENTED_EDGE ( 'NONE', *, *, #31222, .T. ) ;
#19650=DIRECTION ( 'NONE',  ( 0.8660254037844380415, 0.5000000000000011102, 0.000000000000000000 ) ) ;
#19676=ORIENTED_EDGE ( 'NONE', *, *, #33502, .F. ) ;
#19685=LINE ( 'NONE', #42083, #14115 ) ;
#19707=CARTESIAN_POINT ( 'NONE',  ( -24.57312852195785524, 18.34675584111407787, 4.549864924635812713 ) ) ;
#19716=CARTESIAN_POINT ( 'NONE',  ( -56.66762604419704985, 5.055998648713354804, 2.999999999999993339 ) ) ;
#19738=EDGE_CURVE ( 'NONE', #42394, #17567, #20995, .T. ) ;
#19759=CARTESIAN_POINT ( 'NONE',  ( -22.14101869848777682, 19.68270265044663958, 4.490773887887535842 ) ) ;
#19766=EDGE_CURVE ( 'NONE', #39800, #7659, #40360, .T. ) ;
#19778=VECTOR ( 'NONE', #51279, 1000.000000000000000 ) ;
#19819=ORIENTED_EDGE ( 'NONE', *, *, #18218, .F. ) ;
#19849=MECHANICAL_DESIGN_GEOMETRIC_PRESENTATION_REPRESENTATION('',(#32581),#40740);
#19901=VERTEX_POINT ( 'NONE', #45434 ) ;
#19955=CARTESIAN_POINT ( 'NONE',  ( -60.92294909528611413, 7.225036622302098976, 2.999999999999993339 ) ) ;
#19985=VERTEX_POINT ( 'NONE', #8819 ) ;
#20007=EDGE_LOOP ( 'NONE', ( #47045, #54136, #2427, #4044 ) ) ;
#20038=ORIENTED_EDGE ( 'NONE', *, *, #31540, .T. ) ;
#20075=EDGE_LOOP ( 'NONE', ( #44222, #55075, #26109, #38362, #8284, #28341, #45302, #31079, #35192, #7435, #10938, #51437, #614, #1180, #51913, #44400, #54425, #5864, #34421, #3739, #23826, #945, #19037, #9812, #44459, #42235, #54967 ) ) ;
#20155=AXIS2_PLACEMENT_3D ( 'NONE', #36898, #37153, #50202 ) ;
#20187=DIRECTION ( 'NONE',  ( -0.2588190451025212946, -0.9659258262890680902, 0.000000000000000000 ) ) ;
#20253=B_SPLINE_CURVE_WITH_KNOTS ( 'NONE', 3,
 ( #43799, #47220, #4630, #35305 ),
 .UNSPECIFIED., .F., .F.,
 ( 4, 4 ),
 ( 0.0001107606836644239992, 0.0004080808962162847881 ),
 .UNSPECIFIED. ) ;
#20277=CARTESIAN_POINT ( 'NONE',  ( -11.91804826722769306, 25.86399001096056338, -4.999999999999888978 ) ) ;
#20355=DIRECTION ( 'NONE',  ( -0.000000000000000000, -0.000000000000000000, 1.000000000000000000 ) ) ;
#20386=FACE_OUTER_BOUND ( 'NONE', #38282, .T. ) ;
#20417=AXIS2_PLACEMENT_3D ( 'NONE', #32976, #15371, #19650 ) ;
#20429=ORIENTED_EDGE ( 'NONE', *, *, #45981, .T. ) ;
#20446=CARTESIAN_POINT ( 'NONE',  ( -25.98475788909843587, 17.60307238499724392, 4.611630842834720134 ) ) ;
#20475=ORIENTED_EDGE ( 'NONE', *, *, #10308, .F. ) ;
#20496=AXIS2_PLACEMENT_3D ( 'NONE', #1736, #35286, #5193 ) ;
#20503=ORIENTED_EDGE ( 'NONE', *, *, #8674, .T. ) ;
#20596=EDGE_CURVE ( 'NONE', #27675, #460, #45801, .T. ) ;
#20597=CARTESIAN_POINT ( 'NONE',  ( -13.17964512767721530, 23.31695337602389273, -3.677660435020122964 ) ) ;
#20617=EDGE_CURVE ( 'NONE', #7659, #21622, #33708, .T. ) ;
#20618=DIRECTION ( 'NONE',  ( -0.3583679495452925523, -0.9335804264972047406, 0.000000000000000000 ) ) ;
#20638=CARTESIAN_POINT ( 'NONE',  ( -26.23274948935539541, 17.48484997744522929, -4.621578396180252568 ) ) ;
#20685=DIRECTION ( 'NONE',  ( 0.3535533905932752297, -0.6123724356957952475, 0.7071067811865462405 ) ) ;
#20701=PLANE ( 'NONE',  #55433 ) ;
#20707=DIRECTION ( 'NONE',  ( -1.000000000000000000, 0.000000000000000000, 0.000000000000000000 ) ) ;
#20843=CARTESIAN_POINT ( 'NONE',  ( -20.72814514249575168, 20.40220053346460460, -4.343046601173932153 ) ) ;
#20867=CARTESIAN_POINT ( 'NONE',  ( -24.96676581047183063, 18.24370688441070953, 4.565775410814726598 ) ) ;
#20886=CARTESIAN_POINT ( 'NONE',  ( -20.38426584293951294, 20.88941447422692477, 4.312559560550884186 ) ) ;
#20900=ORIENTED_EDGE ( 'NONE', *, *, #4543, .F. ) ;
#20949=CARTESIAN_POINT ( 'NONE',  ( -19.60084266227577032, 19.60967325090364000, 4.310338978832157331 ) ) ;
#20995=B_SPLINE_CURVE_WITH_KNOTS ( 'NONE', 3,
 ( #27879, #31575, #32418, #9719 ),
 .UNSPECIFIED., .F., .F.,
 ( 4, 4 ),
 ( 9.874130977897000849E-05, 0.0003960674641214396866 ),
 .UNSPECIFIED. ) ;
#21031=FACE_OUTER_BOUND ( 'NONE', #8325, .T. ) ;
#21033=FACE_OUTER_BOUND ( 'NONE', #42936, .T. ) ;
#21068=AXIS2_PLACEMENT_3D ( 'NONE', #2573, #2829, #11088 ) ;
#21072=DIRECTION ( 'NONE',  ( 0.9659258262890692004, -0.2588190451025176864, 0.000000000000000000 ) ) ;
#21112=VECTOR ( 'NONE', #675, 1000.000000000000000 ) ;
#21149=DIRECTION ( 'NONE',  ( -0.2588190451025212946, -0.9659258262890680902, 0.000000000000000000 ) ) ;
#21150=UNCERTAINTY_MEASURE_WITH_UNIT (LENGTH_MEASURE( 1.000000000000000082E-05 ), #37557, 'distance_accuracy_value', 'NONE');
#21234=EDGE_CURVE ( 'NONE', #25987, #33400, #22903, .T. ) ;
#21261=ORIENTED_EDGE ( 'NONE', *, *, #10829, .F. ) ;
#21275=VECTOR ( 'NONE', #29926, 1000.000000000000114 ) ;
#21326=CARTESIAN_POINT ( 'NONE',  ( -24.87971537937347932, 18.22038179169711825, 4.563126927700496438 ) ) ;
#21359=CYLINDRICAL_SURFACE ( 'NONE', #45686, 2.000000000000000888 ) ;
#21397=CIRCLE ( 'NONE', #24147, 2.000000000000002220 ) ;
#21448=ADVANCED_FACE ( 'NONE', ( #20386 ), #6494, .F. ) ;
#21461=VECTOR ( 'NONE', #20355, 1000.000000000000000 ) ;
#21500=ADVANCED_FACE ( 'NONE', ( #33720 ), #15846, .F. ) ;
#21504=VERTEX_POINT ( 'NONE', #2763 ) ;
#21533=DIRECTION ( 'NONE',  ( 0.3535533905932738974, -0.6123724356957929160, -0.7071067811865487940 ) ) ;
#21545=B_SPLINE_CURVE_WITH_KNOTS ( 'NONE', 3,
 ( #30041, #51349, #50768, #4222 ),
 .UNSPECIFIED., .F., .F.,
 ( 4, 4 ),
 ( 0.000000000000000000, 0.0003538173816226116894 ),
 .UNSPECIFIED. ) ;
#21620=CARTESIAN_POINT ( 'NONE',  ( -56.20083583094844926, 4.876814673940706335, 2.999999999999993339 ) ) ;
#21622=VERTEX_POINT ( 'NONE', #22075 ) ;
#21631=VERTEX_POINT ( 'NONE', #47344 ) ;
#21647=ORIENTED_EDGE ( 'NONE', *, *, #34493, .T. ) ;
#21670=DIRECTION ( 'NONE',  ( 0.2113248654051873565, 0.7886751345948123104, 0.5773502691896265082 ) ) ;
#21700=LINE ( 'NONE', #373, #35949 ) ;
#21712=CARTESIAN_POINT ( 'NONE',  ( -14.32726051673741452, 22.65437732222383360, -3.841877719209101372 ) ) ;
#21778=FACE_OUTER_BOUND ( 'NONE', #2785, .T. ) ;
#21789=FACE_OUTER_BOUND ( 'NONE', #55274, .T. ) ;
#21796=DIRECTION ( 'NONE',  ( -0.000000000000000000, -0.000000000000000000, 1.000000000000000000 ) ) ;
#21798=CARTESIAN_POINT ( 'NONE',  ( -35.53815943785284759, 10.40825912036386214, -4.912923275970548787 ) ) ;
#21803=CARTESIAN_POINT ( 'NONE',  ( -19.65908866086925144, 19.57604490793647400, 4.314202863308498337 ) ) ;
#21861=LINE ( 'NONE', #9673, #25085 ) ;
#21876=EDGE_LOOP ( 'NONE', ( #35614, #40126, #38572, #39226 ) ) ;
#21954=B_SPLINE_CURVE_WITH_KNOTS ( 'NONE', 3,
 ( #40259, #22936, #14984, #31746 ),
 .UNSPECIFIED., .F., .F.,
 ( 4, 4 ),
 ( 0.000000000000000000, 0.0002393041340872677626 ),
 .UNSPECIFIED. ) ;
#21973=CARTESIAN_POINT ( 'NONE',  ( -22.04728230093569152, 19.65758605842115969, -4.422151119964278010 ) ) ;
#21981=CARTESIAN_POINT ( 'NONE',  ( -23.44701637808619665, 18.93456746265863799, 4.495868649597294819 ) ) ;
#22020=ADVANCED_FACE ( 'NONE', ( #40160 ), #39331, .F. ) ;
#22023=CARTESIAN_POINT ( 'NONE',  ( -46.52156441860518754, 5.799038105676674881, 5.000000000000000000 ) ) ;
#22028=DIRECTION ( 'NONE',  ( -0.000000000000000000, -0.000000000000000000, 1.000000000000000000 ) ) ;
#22071=CARTESIAN_POINT ( 'NONE',  ( -21.93567689722629765, 19.99370688441071309, -4.657437592157546824 ) ) ;
#22075=CARTESIAN_POINT ( 'NONE',  ( -63.56784591066751489, 8.775889882925216767, -3.000000000000000000 ) ) ;
#22077=CARTESIAN_POINT ( 'NONE',  ( -21.06965149344186372, 20.49370688441071664, -4.356725136697556344 ) ) ;
#22081=CARTESIAN_POINT ( 'NONE',  ( -42.10458952830071411, 6.617128940028910833, -4.991983769317021924 ) ) ;
#22103=ADVANCED_FACE ( 'NONE', ( #31663 ), #18291, .F. ) ;
#22146=CARTESIAN_POINT ( 'NONE',  ( -22.02230563637845151, 19.67040402849924163, -4.420763475398227449 ) ) ;
#22209=VECTOR ( 'NONE', #47465, 1000.000000000000000 ) ;
#22255=CARTESIAN_POINT ( 'NONE',  ( -24.53375310857961367, 18.49370688441070953, 4.657440554554202805 ) ) ;
#22278=ORIENTED_EDGE ( 'NONE', *, *, #55662, .T. ) ;
#22282=AXIS2_PLACEMENT_3D ( 'NONE', #21620, #8256, #56236 ) ;
#22305=DIRECTION ( 'NONE',  ( 1.000000000000000000, 0.000000000000000000, 0.000000000000000000 ) ) ;
#22311=VECTOR ( 'NONE', #22658, 1000.000000000000000 ) ;
#22328=CARTESIAN_POINT ( 'NONE',  ( -22.36868959911851462, 19.74370688441071309, -4.657437592157546824 ) ) ;
#22334=CARTESIAN_POINT ( 'NONE',  ( -21.06965149344186372, 20.49370688441071664, -4.356725136697556344 ) ) ;
#22353=CIRCLE ( 'NONE', #29605, 0.5000000000000004441 ) ;
#22387=CARTESIAN_POINT ( 'NONE',  ( -15.88066920543382921, 21.75751639764346024, -4.011138004292909898 ) ) ;
#22455=CARTESIAN_POINT ( 'NONE',  ( -50.45472955569960760, 3.742236127018431890, 5.000000000000000000 ) ) ;
#22467=CARTESIAN_POINT ( 'NONE',  ( -64.10539783498545319, 7.375519243179410545, 5.000000000000000000 ) ) ;
#22472=DIRECTION ( 'NONE',  ( -0.000000000000000000, 0.000000000000000000, -1.000000000000000000 ) ) ;
#22537=LINE ( 'NONE', #14561, #16981 ) ;
#22575=EDGE_LOOP ( 'NONE', ( #13937, #19676, #31429, #24985, #44160, #29858 ) ) ;
#22597=ORIENTED_EDGE ( 'NONE', *, *, #20617, .T. ) ;
#22618=CARTESIAN_POINT ( 'NONE',  ( -19.39860431275360853, 21.26603824944626808, -4.250162336171596777 ) ) ;
#22643=DIRECTION ( 'NONE',  ( 0.9335804264972041855, -0.3583679495452941066, 0.000000000000000000 ) ) ;
#22658=DIRECTION ( 'NONE',  ( -0.000000000000000000, -0.000000000000000000, 1.000000000000000000 ) ) ;
#22660=ADVANCED_FACE ( 'NONE', ( #12156 ), #29191, .F. ) ;
#22670=VERTEX_POINT ( 'NONE', #15854 ) ;
#22707=SHAPE_REPRESENTATION_RELATIONSHIP ( 'NONE' , 'NONE' ,  #24540, #27288 ) ;
#22718=ORIENTED_EDGE ( 'NONE', *, *, #45981, .F. ) ;
#22787=CARTESIAN_POINT ( 'NONE',  ( -23.59415828741828136, 18.97399401843694022, -4.500635383149576896 ) ) ;
#22878=ORIENTED_EDGE ( 'NONE', *, *, #42845, .T. ) ;
#22903=CIRCLE ( 'NONE', #31940, 2.000000000000002220 ) ;
#22935=CARTESIAN_POINT ( 'NONE',  ( -27.34714091995699548, 16.86939667417711775, 4.665742070404716557 ) ) ;
#22936=CARTESIAN_POINT ( 'NONE',  ( -23.25534986176962704, 19.16669654271327161, 4.483237965442247841 ) ) ;
#22974=DIRECTION ( 'NONE',  ( -0.2588190451025176864, -0.9659258262890692004, 0.000000000000000000 ) ) ;
#22984=CARTESIAN_POINT ( 'NONE',  ( -20.69764258542294399, 20.51603762622111304, 4.338448882013300256 ) ) ;
#22988=CARTESIAN_POINT ( 'NONE',  ( -11.88054826722768276, 25.79903810567671130, 5.000000000000000000 ) ) ;
#23041=ORIENTED_EDGE ( 'NONE', *, *, #18197, .T. ) ;
#23056=CYLINDRICAL_SURFACE ( 'NONE', #20496, 0.5000000000000004441 ) ;
#23080=LINE ( 'NONE', #919, #11046 ) ;
#23086=CARTESIAN_POINT ( 'NONE',  ( -61.70068505767310540, 8.059153983834628221, 5.000000000000000000 ) ) ;
#23160=CARTESIAN_POINT ( 'NONE',  ( -16.20482545075801895, 23.30241550971489772, -3.967651922502964723 ) ) ;
#23165=CARTESIAN_POINT ( 'NONE',  ( -20.57714959317112147, 20.77805298910839582, -4.325263209797152619 ) ) ;
#23214=ORIENTED_EDGE ( 'NONE', *, *, #12341, .F. ) ;
#23227=CARTESIAN_POINT ( 'NONE',  ( -39.55045063245202641, 8.091761719094847649, 5.000000000000000000 ) ) ;
#23257=LINE ( 'NONE', #23784, #5696 ) ;
#23266=CARTESIAN_POINT ( 'NONE',  ( -50.02554558092695913, 3.776013638374817294, 5.000000000000000000 ) ) ;
#23270=CARTESIAN_POINT ( 'NONE',  ( -46.00906441860568918, 4.911362066797304138, 5.000000000000000000 ) ) ;
#23288=CARTESIAN_POINT ( 'NONE',  ( -11.63054826722768453, 25.36602540378449433, 3.000000000000000000 ) ) ;
#23297=CARTESIAN_POINT ( 'NONE',  ( -62.23823698199103660, 6.658783344088824663, 5.000000000000000000 ) ) ;
#23369=CARTESIAN_POINT ( 'NONE',  ( -23.44702061269273230, 18.93456859731804087, -4.495868787147773382 ) ) ;
#23385=FACE_OUTER_BOUND ( 'NONE', #17761, .T. ) ;
#23389=DIRECTION ( 'NONE',  ( -0.000000000000000000, -0.000000000000000000, -1.000000000000000000 ) ) ;
#23443=EDGE_CURVE ( 'NONE', #21504, #41243, #13517, .T. ) ;
#23445=CARTESIAN_POINT ( 'NONE',  ( -20.33106256009199697, 20.92013140390070802, -4.309024953547888614 ) ) ;
#23459=CARTESIAN_POINT ( 'NONE',  ( -46.52156441860518754, 5.799038105676674881, 5.000000000000000000 ) ) ;
#23462=CARTESIAN_POINT ( 'NONE',  ( -19.42910703681909368, 21.15220053346460816, -4.657437592157546824 ) ) ;
#23471=CARTESIAN_POINT ( 'NONE',  ( -23.44702061269273230, 18.93456859731804087, -4.495868787147773382 ) ) ;
#23544=LINE ( 'NONE', #28346, #17798 ) ;
#23550=SURFACE_STYLE_USAGE ( .BOTH. , #14220 ) ;
#23615=FACE_OUTER_BOUND ( 'NONE', #9390, .T. ) ;
#23623=CARTESIAN_POINT ( 'NONE',  ( -24.56000265080053069, 18.39574225916684824, -4.548402510131950294 ) ) ;
#23662=CARTESIAN_POINT ( 'NONE',  ( -24.96676581047183063, 18.24370688441070953, -4.565775476651154463 ) ) ;
#23722=ORIENTED_EDGE ( 'NONE', *, *, #32393, .F. ) ;
#23746=AXIS2_PLACEMENT_3D ( 'NONE', #50630, #54886, #25084 ) ;
#23784=CARTESIAN_POINT ( 'NONE',  ( -24.53375310857961367, 18.49370688441070953, -4.657437592157546824 ) ) ;
#23795=DIRECTION ( 'NONE',  ( 0.000000000000000000, 0.000000000000000000, 1.000000000000000000 ) ) ;
#23819=LINE ( 'NONE', #54758, #9661 ) ;
#23826=ORIENTED_EDGE ( 'NONE', *, *, #10829, .T. ) ;
#23870=ORIENTED_EDGE ( 'NONE', *, *, #47402, .F. ) ;
#23871=DIRECTION ( 'NONE',  ( 1.000000000000000000, -3.469446951953611033E-15, 0.000000000000000000 ) ) ;
#23903=ORIENTED_EDGE ( 'NONE', *, *, #48168, .T. ) ;
#23953=EDGE_LOOP ( 'NONE', ( #27996, #41051, #40055, #13725, #11295, #21261 ) ) ;
#23986=CARTESIAN_POINT ( 'NONE',  ( -45.73406441860519323, 4.435048094716153244, -5.000000000000000000 ) ) ;
#24024=AXIS2_PLACEMENT_3D ( 'NONE', #45189, #11377, #40655 ) ;
#24120=VECTOR ( 'NONE', #50650, 1000.000000000000000 ) ;
#24147=AXIS2_PLACEMENT_3D ( 'NONE', #33041, #36454, #24502 ) ;
#24159=VERTEX_POINT ( 'NONE', #48736 ) ;
#24168=AXIS2_PLACEMENT_3D ( 'NONE', #48641, #53709, #35562 ) ;
#24210=LINE ( 'NONE', #32172, #12384 ) ;
#24230=CARTESIAN_POINT ( 'NONE',  ( -56.70083583094844926, 4.876814673940706335, 2.999999999999993339 ) ) ;
#24231=ORIENTED_EDGE ( 'NONE', *, *, #47402, .T. ) ;
#24268=PLANE ( 'NONE',  #43338 ) ;
#24370=CARTESIAN_POINT ( 'NONE',  ( -20.72814514249575168, 20.40220053346460460, 4.343046601168861542 ) ) ;
#24390=EDGE_LOOP ( 'NONE', ( #8797, #54606, #18568, #30013, #30678, #33840 ) ) ;
#24420=B_SPLINE_CURVE_WITH_KNOTS ( 'NONE', 3,
 ( #1943, #23288, #6505, #32621 ),
 .UNSPECIFIED., .F., .F.,
 ( 4, 4 ),
 ( 0.000000000000000000, 1.000000000000000000 ),
 .UNSPECIFIED. ) ;
#24502=DIRECTION ( 'NONE',  ( 0.9335804264972044075, -0.3583679495452936070, 0.000000000000000000 ) ) ;
#24540=SHAPE_REPRESENTATION ( 'Upper Lever Press Arm', ( #2610 ), #44334 ) ;
#24541=VERTEX_POINT ( 'NONE', #48932 ) ;
#24554=CARTESIAN_POINT ( 'NONE',  ( -50.02554558092695913, 3.776013638374817294, 5.000000000000000000 ) ) ;
#24562=UNCERTAINTY_MEASURE_WITH_UNIT (LENGTH_MEASURE( 1.000000000000000082E-05 ), #48842, 'distance_accuracy_value', 'NONE');
#24607=ORIENTED_EDGE ( 'NONE', *, *, #16790, .T. ) ;
#24617=VERTEX_POINT ( 'NONE', #27634 ) ;
#24651=CARTESIAN_POINT ( 'NONE',  ( -49.27554558092695913, 2.476975532698160620, 5.000000000000000000 ) ) ;
#24670=EDGE_CURVE ( 'NONE', #33400, #7659, #45770, .T. ) ;
#24688=ORIENTED_EDGE ( 'NONE', *, *, #12515, .F. ) ;
#24735=DIRECTION ( 'NONE',  ( -0.000000000000000000, -0.000000000000000000, -1.000000000000000000 ) ) ;
#24765=CARTESIAN_POINT ( 'NONE',  ( -23.66772770479517618, 18.99370688441070953, -4.657437592157546824 ) ) ;
#24826=CARTESIAN_POINT ( 'NONE',  ( -61.38973930853472183, 7.404220597074748333, 2.999999999999993339 ) ) ;
#24844=CARTESIAN_POINT ( 'NONE',  ( -26.26580391614848864, 17.49370688441070953, -4.657437592157546824 ) ) ;
#24862=AXIS2_PLACEMENT_3D ( 'NONE', #25060, #55999, #17093 ) ;
#24863=CARTESIAN_POINT ( 'NONE',  ( -22.04727804374295275, 19.65758491770980143, 4.422150965879553475 ) ) ;
#24884=B_SPLINE_CURVE_WITH_KNOTS ( 'NONE', 3,
 ( #41515, #32694, #33541, #45755 ),
 .UNSPECIFIED., .F., .F.,
 ( 4, 4 ),
 ( 0.000000000000000000, 7.270906544745860773E-05 ),
 .UNSPECIFIED. ) ;
#24888=CARTESIAN_POINT ( 'NONE',  ( -13.00639936336226476, 25.14902767225597913, -3.505746236942866911 ) ) ;
#24972=VECTOR ( 'NONE', #17583, 1000.000000000000000 ) ;
#24985=ORIENTED_EDGE ( 'NONE', *, *, #26082, .T. ) ;
#25060=CARTESIAN_POINT ( 'NONE',  ( -24.96676581047183063, 18.24370688441070953, -4.657437592157546824 ) ) ;
#25084=DIRECTION ( 'NONE',  ( 0.9335804264972044075, -0.3583679495452936070, 8.673617379884025611E-16 ) ) ;
#25085=VECTOR ( 'NONE', #52792, 1000.000000000000000 ) ;
#25142=VERTEX_POINT ( 'NONE', #15072 ) ;
#25154=DIRECTION ( 'NONE',  ( -0.3583679495452941066, -0.9335804264972041855, 0.000000000000000000 ) ) ;
#25260=EDGE_CURVE ( 'NONE', #34711, #22670, #25824, .T. ) ;
#25268=ORIENTED_EDGE ( 'NONE', *, *, #49320, .T. ) ;
#25312=CARTESIAN_POINT ( 'NONE',  ( -50.02554558092695913, 3.776013638374815962, 5.000000000000000000 ) ) ;
#25370=CARTESIAN_POINT ( 'NONE',  ( -21.93567689722629765, 19.99370688441071309, 4.408989160011352659 ) ) ;
#25411=CARTESIAN_POINT ( 'NONE',  ( -50.02554558092695913, 3.776013638374817294, 5.000000000000000000 ) ) ;
#25414=EDGE_CURVE ( 'NONE', #12684, #42224, #36292, .T. ) ;
#25435=CARTESIAN_POINT ( 'NONE',  ( -56.48844206942440138, 5.522788861961955398, 2.999999999999993339 ) ) ;
#25512=ORIENTED_EDGE ( 'NONE', *, *, #31540, .F. ) ;
#25519=ORIENTED_EDGE ( 'NONE', *, *, #33502, .T. ) ;
#25568=CARTESIAN_POINT ( 'NONE',  ( -50.45472955569960760, 3.742236127018431890, -5.000000000000000000 ) ) ;
#25642=ORIENTED_EDGE ( 'NONE', *, *, #19738, .T. ) ;
#25679=CARTESIAN_POINT ( 'NONE',  ( -13.72345201801339165, 23.00298632150112255, -3.759965536548706133 ) ) ;
#25680=EDGE_LOOP ( 'NONE', ( #37878, #53814, #39047, #36632 ) ) ;
#25774=FACE_OUTER_BOUND ( 'NONE', #10460, .T. ) ;
#25795=CARTESIAN_POINT ( 'NONE',  ( -28.01304021813471934, 14.75288872755216119, 4.717228875401151988 ) ) ;
#25824=LINE ( 'NONE', #30903, #45742 ) ;
#25941=CARTESIAN_POINT ( 'NONE',  ( -21.93567689722629765, 19.99370688441071309, 4.657440554554202805 ) ) ;
#25944=CARTESIAN_POINT ( 'NONE',  ( -27.13182931993292257, 16.99370688441070953, -4.657437592157546824 ) ) ;
#25958=CARTESIAN_POINT ( 'NONE',  ( -11.88054826722768276, 25.79903810567671130, 3.000000000000000888 ) ) ;
#25987=VERTEX_POINT ( 'NONE', #34412 ) ;
#26000=ORIENTED_EDGE ( 'NONE', *, *, #518, .F. ) ;
#26007=EDGE_CURVE ( 'NONE', #44683, #46842, #11965, .T. ) ;
#26021=CARTESIAN_POINT ( 'NONE',  ( -23.23471500290295921, 19.24370688441070953, 4.480778704491060971 ) ) ;
#26082=EDGE_CURVE ( 'NONE', #10688, #4495, #13942, .T. ) ;
#26087=CARTESIAN_POINT ( 'NONE',  ( -28.37605857990474334, 14.54329997866345714, -4.729543700631310799 ) ) ;
#26109=ORIENTED_EDGE ( 'NONE', *, *, #1552, .T. ) ;
#26138=FACE_OUTER_BOUND ( 'NONE', #4011, .T. ) ;
#26181=CARTESIAN_POINT ( 'NONE',  ( -61.52150108290046404, 8.525944197083212828, -3.000000000000000000 ) ) ;
#26186=ORIENTED_EDGE ( 'NONE', *, *, #9859, .T. ) ;
#26208=CARTESIAN_POINT ( 'NONE',  ( -26.09471150760941072, 17.54484258725233659, -4.616176205589227699 ) ) ;
#26237=ADVANCED_FACE ( 'NONE', ( #15341 ), #53672, .F. ) ;
#26243=CARTESIAN_POINT ( 'NONE',  ( -11.43872127411717443, 24.32207623151542464, -3.308936884429647840 ) ) ;
#26284=CARTESIAN_POINT ( 'NONE',  ( -13.94269994003180457, 24.60845428227341003, -3.679749630833339946 ) ) ;
#26288=LINE ( 'NONE', #4708, #38713 ) ;
#26295=ORIENTED_EDGE ( 'NONE', *, *, #52184, .F. ) ;
#26299=ORIENTED_EDGE ( 'NONE', *, *, #44338, .T. ) ;
#26335=CARTESIAN_POINT ( 'NONE',  ( -58.57533928340691887, 0.08623575067603483912, 2.999999999999993339 ) ) ;
#26337=ORIENTED_EDGE ( 'NONE', *, *, #455, .T. ) ;
#26545=CARTESIAN_POINT ( 'NONE',  ( -61.38973930853472183, 7.404220597074748333, 2.999999999999993339 ) ) ;
#26555=CARTESIAN_POINT ( 'NONE',  ( -56.48844206942440138, 5.522788861961955398, -3.000000000000007105 ) ) ;
#26616=CARTESIAN_POINT ( 'NONE',  ( -28.51944453287105219, 14.46051606012035151, -4.734328798303309327 ) ) ;
#26676=EDGE_CURVE ( 'NONE', #36742, #40396, #47866, .T. ) ;
#26692=AXIS2_PLACEMENT_3D ( 'NONE', #42724, #3823, #21149 ) ;
#26706=FACE_OUTER_BOUND ( 'NONE', #28050, .T. ) ;
#26779=CARTESIAN_POINT ( 'NONE',  ( -11.13054826722768098, 24.50000000000005684, -3.000000000000000000 ) ) ;
#26785=DIRECTION ( 'NONE',  ( -1.000000000000000000, 0.000000000000000000, -0.000000000000000000 ) ) ;
#26800=VECTOR ( 'NONE', #21670, 1000.000000000000000 ) ;
#26825=EDGE_CURVE ( 'NONE', #52748, #40704, #32828, .T. ) ;
#26846=CYLINDRICAL_SURFACE ( 'NONE', #1456, 0.5000000000000004441 ) ;
#26859=CARTESIAN_POINT ( 'NONE',  ( -13.04051704107165399, 25.12932982184632635, -3.513244100307224116 ) ) ;
#26878=EDGE_LOOP ( 'NONE', ( #28769, #4066, #8999, #15220, #55223, #35442 ) ) ;
#26888=VECTOR ( 'NONE', #37083, 1000.000000000000114 ) ;
#26924=CARTESIAN_POINT ( 'NONE',  ( -28.40705682302959900, 14.52540313465091160, -4.730581911476714474 ) ) ;
#26935=CARTESIAN_POINT ( 'NONE',  ( -56.02165185617580079, 5.343604887189308705, -3.000000000000007105 ) ) ;
#26953=VERTEX_POINT ( 'NONE', #16261 ) ;
#26989=ORIENTED_EDGE ( 'NONE', *, *, #7444, .T. ) ;
#27083=ORIENTED_EDGE ( 'NONE', *, *, #4499, .T. ) ;
#27097=CARTESIAN_POINT ( 'NONE',  ( -11.88054826722768276, 25.79903810567671130, 3.000000000000000888 ) ) ;
#27103=VERTEX_POINT ( 'NONE', #4354 ) ;
#27107=CARTESIAN_POINT ( 'NONE',  ( -22.36868959911851462, 19.74370688441071309, -4.657437592157546824 ) ) ;
#27113=CARTESIAN_POINT ( 'NONE',  ( -21.06965149344186372, 20.49370688441071664, -4.657437592157546824 ) ) ;
#27180=LINE ( 'NONE', #44781, #5452 ) ;
#27182=CARTESIAN_POINT ( 'NONE',  ( -28.38032086473889137, 14.54083914736709993, -4.729686555805564296 ) ) ;
#27235=CARTESIAN_POINT ( 'NONE',  ( -46.02156441860540781, 4.933012701892111274, -5.000000000000000000 ) ) ;
#27250=EDGE_CURVE ( 'NONE', #22670, #39800, #15589, .T. ) ;
#27262=ORIENTED_EDGE ( 'NONE', *, *, #37372, .F. ) ;
#27281=ORIENTED_EDGE ( 'NONE', *, *, #33406, .F. ) ;
#27288=ADVANCED_BREP_SHAPE_REPRESENTATION ( '', ( #41257, #2610 ), #44334 ) ;
#27303=DIRECTION ( 'NONE',  ( 0.9659258262890692004, -0.2588190451025176864, 0.000000000000000000 ) ) ;
#27312=VECTOR ( 'NONE', #48193, 1000.000000000000000 ) ;
#27367=ADVANCED_FACE ( 'NONE', ( #46026 ), #2296, .F. ) ;
#27377=CARTESIAN_POINT ( 'NONE',  ( -20.72814514249575168, 20.40220053346460460, 4.343046601168861542 ) ) ;
#27398=CARTESIAN_POINT ( 'NONE',  ( -16.32483125059555107, 23.23313012887437168, -3.980127950647806223 ) ) ;
#27407=CARTESIAN_POINT ( 'NONE',  ( -21.35351436783577483, 20.32981857746640841, -4.374509389852473618 ) ) ;
#27432=EDGE_LOOP ( 'NONE', ( #16501, #19531, #18926, #36169, #42573, #54009 ) ) ;
#27471=CARTESIAN_POINT ( 'NONE',  ( -19.33759994122731385, 21.49370731433205250, -4.239680377485293583 ) ) ;
#27488=ORIENTED_EDGE ( 'NONE', *, *, #24670, .T. ) ;
#27524=DIRECTION ( 'NONE',  ( -0.7886751345948130876, 0.2113248654051844977, -0.5773502691896263972 ) ) ;
#27611=PLANE ( 'NONE',  #20417 ) ;
#27634=CARTESIAN_POINT ( 'NONE',  ( -60.88973930853472893, 7.404220597074750110, -3.000000000000006661 ) ) ;
#27653=ORIENTED_EDGE ( 'NONE', *, *, #42331, .F. ) ;
#27661=CARTESIAN_POINT ( 'NONE',  ( -21.35352775840775408, 20.32981084641607339, 4.374505632834054580 ) ) ;
#27671=VERTEX_POINT ( 'NONE', #24370 ) ;
#27675=VERTEX_POINT ( 'NONE', #41681 ) ;
#27690=ADVANCED_FACE ( 'NONE', ( #49674 ), #28646, .F. ) ;
#27719=CARTESIAN_POINT ( 'NONE',  ( -32.96103433568752195, 13.62821379940322508, 4.845353415783987927 ) ) ;
#27781=VECTOR ( 'NONE', #41968, 1000.000000000000114 ) ;
#27812=DIRECTION ( 'NONE',  ( 0.5000000000000011102, -0.8660254037844380415, 0.000000000000000000 ) ) ;
#27817=CARTESIAN_POINT ( 'NONE',  ( -11.09304826722767956, 24.43504809471621542, 3.000000000000000000 ) ) ;
#27857=EDGE_CURVE ( 'NONE', #27103, #27945, #21545, .T. ) ;
#27879=CARTESIAN_POINT ( 'NONE',  ( -24.83619454210204580, 18.20872041849631984, -4.561852789702152577 ) ) ;
#27940=CARTESIAN_POINT ( 'NONE',  ( -27.56484202182514665, 16.74370688441070953, -4.657437592157546824 ) ) ;
#27945=VERTEX_POINT ( 'NONE', #22077 ) ;
#27946=CARTESIAN_POINT ( 'NONE',  ( -19.33760068587298164, 21.49370688441072019, 4.239878526350478793 ) ) ;
#27954=ORIENTED_EDGE ( 'NONE', *, *, #25260, .F. ) ;
#27996=ORIENTED_EDGE ( 'NONE', *, *, #48168, .F. ) ;
#28018=CARTESIAN_POINT ( 'NONE',  ( -19.42910703681909368, 21.15220053346460816, -4.255330291692488665 ) ) ;
#28041=ADVANCED_FACE ( 'NONE', ( #1039, #48477 ), #52181, .F. ) ;
#28049=ORIENTED_EDGE ( 'NONE', *, *, #16723, .F. ) ;
#28050=EDGE_LOOP ( 'NONE', ( #13310, #27488, #6723, #47580, #27954, #16654, #688, #9175 ) ) ;
#28186=DIRECTION ( 'NONE',  ( -1.000000000000000000, 0.000000000000000000, 0.000000000000000000 ) ) ;
#28205=LINE ( 'NONE', #50050, #33074 ) ;
#28208=CARTESIAN_POINT ( 'NONE',  ( -24.54687820731135162, 18.44472334908947175, 4.546935074492525430 ) ) ;
#28241=CARTESIAN_POINT ( 'NONE',  ( -22.02230666951336246, 19.67040017278726438, 4.420763615217817133 ) ) ;
#28265=CARTESIAN_POINT ( 'NONE',  ( -56.20083583094844926, 4.876814673940706335, -3.000000000000007105 ) ) ;
#28267=ORIENTED_EDGE ( 'NONE', *, *, #37009, .F. ) ;
#28275=EDGE_CURVE ( 'NONE', #9690, #37705, #8612, .T. ) ;
#28286=CARTESIAN_POINT ( 'NONE',  ( -24.96676581047183063, 18.24370688441070953, -4.565775476651154463 ) ) ;
#28335=CARTESIAN_POINT ( 'NONE',  ( -11.09304826722767956, 24.43504809471621186, 5.000000000000000888 ) ) ;
#28341=ORIENTED_EDGE ( 'NONE', *, *, #48391, .F. ) ;
#28346=CARTESIAN_POINT ( 'NONE',  ( -20.63663879154963965, 20.74370688441071664, -4.657437592157546824 ) ) ;
#28429=VECTOR ( 'NONE', #24735, 1000.000000000000000 ) ;
#28517=ORIENTED_EDGE ( 'NONE', *, *, #17573, .F. ) ;
#28560=VECTOR ( 'NONE', #10569, 1000.000000000000000 ) ;
#28561=CARTESIAN_POINT ( 'NONE',  ( -27.56453817542467633, 16.74388231021177020, -4.674278956779107652 ) ) ;
#28564=AXIS2_PLACEMENT_3D ( 'NONE', #35021, #17122, #51744 ) ;
#28636=CARTESIAN_POINT ( 'NONE',  ( -11.64304826722767672, 25.38767603887909985, 3.000000000000000000 ) ) ;
#28646=PLANE ( 'NONE',  #41061 ) ;
#28680=EDGE_CURVE ( 'NONE', #682, #24541, #16685, .T. ) ;
#28687=VECTOR ( 'NONE', #47731, 999.9999999999998863 ) ;
#28738=ORIENTED_EDGE ( 'NONE', *, *, #49513, .T. ) ;
#28766=ORIENTED_EDGE ( 'NONE', *, *, #18218, .T. ) ;
#28769=ORIENTED_EDGE ( 'NONE', *, *, #39714, .T. ) ;
#28782=B_SPLINE_CURVE_WITH_KNOTS ( 'NONE', 3,
 ( #968, #18292, #40738, #27377 ),
 .UNSPECIFIED., .F., .F.,
 ( 4, 4 ),
 ( 0.000000000000000000, 0.0003538173816227488952 ),
 .UNSPECIFIED. ) ;
#28846=FACE_OUTER_BOUND ( 'NONE', #45694, .T. ) ;
#28855=CARTESIAN_POINT ( 'NONE',  ( -29.31353752332232077, 15.73409706589058388, -4.735829944523183954 ) ) ;
#28883=CARTESIAN_POINT ( 'NONE',  ( -21.96455318448683514, 19.88593911322026742, 4.412914703902076852 ) ) ;
#28900=ORIENTED_EDGE ( 'NONE', *, *, #9773, .T. ) ;
#28912=EDGE_CURVE ( 'NONE', #21622, #25987, #11325, .T. ) ;
#28920=DIRECTION ( 'NONE',  ( 0.3535533905932738974, -0.6123724356957929160, -0.7071067811865487940 ) ) ;
#29011=EDGE_CURVE ( 'NONE', #53934, #3513, #33679, .T. ) ;
#29029=DIRECTION ( 'NONE',  ( 0.8660254037844380415, 0.5000000000000011102, 0.000000000000000000 ) ) ;
#29079=CARTESIAN_POINT ( 'NONE',  ( -11.64304826723200570, 25.38767603887662716, -5.000000000092198249 ) ) ;
#29099=FACE_OUTER_BOUND ( 'NONE', #47013, .T. ) ;
#29123=B_SPLINE_CURVE_WITH_KNOTS ( 'NONE', 3,
 ( #54014, #23623, #41227, #10849 ),
 .UNSPECIFIED., .F., .F.,
 ( 4, 4 ),
 ( 0.0002015054463949536242, 0.0003537000219815807046 ),
 .UNSPECIFIED. ) ;
#29135=CARTESIAN_POINT ( 'NONE',  ( -12.97875704852626022, 25.16498697016756836, -3.499616475124794679 ) ) ;
#29191=PLANE ( 'NONE',  #42015 ) ;
#29222=EDGE_CURVE ( 'NONE', #12684, #11612, #16089, .T. ) ;
#29227=ADVANCED_FACE ( 'NONE', ( #37107 ), #45090, .T. ) ;
#29283=EDGE_LOOP ( 'NONE', ( #33149, #16027, #23214, #914 ) ) ;
#29349=CARTESIAN_POINT ( 'NONE',  ( -26.21622229497770817, 17.48042152905857449, -4.621141326338904065 ) ) ;
#29376=ORIENTED_EDGE ( 'NONE', *, *, #28912, .T. ) ;
#29439=EDGE_CURVE ( 'NONE', #17024, #9917, #47028, .T. ) ;
#29457=AXIS2_PLACEMENT_3D ( 'NONE', #5949, #23795, #45956 ) ;
#29495=CARTESIAN_POINT ( 'NONE',  ( -23.32622135384906770, 18.90220053346460460, -4.657437592157546824 ) ) ;
#29496=CARTESIAN_POINT ( 'NONE',  ( -20.93015866917345846, 18.84219229648318716, 4.398249846736207225 ) ) ;
#29547=ORIENTED_EDGE ( 'NONE', *, *, #52184, .T. ) ;
#29586=CARTESIAN_POINT ( 'NONE',  ( -25.83906152351308450, 17.72030577168507648, -4.604772726025884388 ) ) ;
#29605=AXIS2_PLACEMENT_3D ( 'NONE', #28265, #32802, #54964 ) ;
#29660=CARTESIAN_POINT ( 'NONE',  ( -63.56784591066751489, 8.775889882925216767, 3.000000000000000000 ) ) ;
#29664=ORIENTED_EDGE ( 'NONE', *, *, #19165, .F. ) ;
#29699=CARTESIAN_POINT ( 'NONE',  ( -21.06965149344186372, 20.49370688441071664, 4.356723378946029790 ) ) ;
#29733=CARTESIAN_POINT ( 'NONE',  ( -26.26580391614848864, 17.49370688441070953, -4.622528711259356271 ) ) ;
#29767=VECTOR ( 'NONE', #27524, 1000.000000000000114 ) ;
#29770=CARTESIAN_POINT ( 'NONE',  ( -25.83279121425626812, 17.74370688441070953, 4.604227610039242968 ) ) ;
#29807=EDGE_LOOP ( 'NONE', ( #2713, #32988, #23870, #31994 ) ) ;
#29855=VERTEX_POINT ( 'NONE', #4629 ) ;
#29856=FACE_OUTER_BOUND ( 'NONE', #25680, .T. ) ;
#29858=ORIENTED_EDGE ( 'NONE', *, *, #3718, .F. ) ;
#29866=ORIENTED_EDGE ( 'NONE', *, *, #53458, .T. ) ;
#29926=DIRECTION ( 'NONE',  ( -0.7886751345948130876, 0.2113248654051844977, 0.5773502691896263972 ) ) ;
#29937=ORIENTED_EDGE ( 'NONE', *, *, #13980, .F. ) ;
#29941=ORIENTED_EDGE ( 'NONE', *, *, #5711, .F. ) ;
#29988=ORIENTED_EDGE ( 'NONE', *, *, #19434, .T. ) ;
#30013=ORIENTED_EDGE ( 'NONE', *, *, #26007, .T. ) ;
#30041=CARTESIAN_POINT ( 'NONE',  ( -20.72814514249575168, 20.40220053346460460, -4.343046601173932153 ) ) ;
#30051=CARTESIAN_POINT ( 'NONE',  ( -12.20289707257236422, 23.88087912856912354, 3.602352073755655137 ) ) ;
#30071=PLANE ( 'NONE',  #2432 ) ;
#30108=( LENGTH_UNIT ( ) NAMED_UNIT ( * ) SI_UNIT ( .MILLI., .METRE. ) );
#30117=CARTESIAN_POINT ( 'NONE',  ( -64.10539783498545319, 7.375519243179410545, 5.000000000000000000 ) ) ;
#30162=AXIS2_PLACEMENT_3D ( 'NONE', #9597, #47929, #22643 ) ;
#30232=ORIENTED_EDGE ( 'NONE', *, *, #20596, .F. ) ;
#30287=EDGE_CURVE ( 'NONE', #46842, #6581, #47007, .T. ) ;
#30288=ORIENTED_EDGE ( 'NONE', *, *, #15082, .F. ) ;
#30393=CARTESIAN_POINT ( 'NONE',  ( -45.77156441860525149, 4.499999999999981348, -5.000000000000000000 ) ) ;
#30413=CARTESIAN_POINT ( 'NONE',  ( -23.27598415104352014, 19.08968832676502458, -4.485782677847319100 ) ) ;
#30528=CARTESIAN_POINT ( 'NONE',  ( -13.30581722938317846, 23.24410787913973664, -3.697606465566034561 ) ) ;
#30542=VERTEX_POINT ( 'NONE', #24863 ) ;
#30630=CARTESIAN_POINT ( 'NONE',  ( -37.22581621634162019, 9.433890025003661250, -4.938189955668043751 ) ) ;
#30677=PLANE ( 'NONE',  #50245 ) ;
#30678=ORIENTED_EDGE ( 'NONE', *, *, #50679, .T. ) ;
#30686=FACE_OUTER_BOUND ( 'NONE', #15988, .T. ) ;
#30699=CARTESIAN_POINT ( 'NONE',  ( -23.25534951586139343, 19.16669783366043589, -4.483237922539919929 ) ) ;
#30721=EDGE_CURVE ( 'NONE', #14093, #682, #36751, .T. ) ;
#30777=DIRECTION ( 'NONE',  ( 0.000000000000000000, 0.000000000000000000, -1.000000000000000000 ) ) ;
#30791=EDGE_CURVE ( 'NONE', #34450, #25142, #42156, .T. ) ;
#30831=CARTESIAN_POINT ( 'NONE',  ( -13.93438848177649092, 24.61325290493446616, -3.678420148561327707 ) ) ;
#30876=CARTESIAN_POINT ( 'NONE',  ( -18.83741502687287905, 20.05043840171031633, -4.259863338787211795 ) ) ;
#30903=CARTESIAN_POINT ( 'NONE',  ( -50.02554558092695913, 3.776013638374817294, -5.000000000000000000 ) ) ;
#30957=VERTEX_POINT ( 'NONE', #3503 ) ;
#30975=ORIENTED_EDGE ( 'NONE', *, *, #43733, .T. ) ;
#31038=EDGE_CURVE ( 'NONE', #54725, #54555, #47800, .T. ) ;
#31051=EDGE_CURVE ( 'NONE', #32191, #48518, #50372, .T. ) ;
#31053=DIRECTION ( 'NONE',  ( -0.7886751345948130876, 0.2113248654051844977, -0.5773502691896263972 ) ) ;
#31077=CARTESIAN_POINT ( 'NONE',  ( -25.83279121425626812, 17.74370688441070953, -4.657437592157546824 ) ) ;
#31079=ORIENTED_EDGE ( 'NONE', *, *, #29011, .F. ) ;
#31104=DIRECTION ( 'NONE',  ( -0.000000000000000000, -0.000000000000000000, -1.000000000000000000 ) ) ;
#31196=CYLINDRICAL_SURFACE ( 'NONE', #49969, 2.000000000000001776 ) ;
#31222=EDGE_CURVE ( 'NONE', #38353, #24617, #5045, .T. ) ;
#31244=DIRECTION ( 'NONE',  ( -0.9335804264972047406, 0.3583679495452925523, 0.000000000000000000 ) ) ;
#31363=CARTESIAN_POINT ( 'NONE',  ( -23.34675815411524979, 18.98665190278753556, 4.490845985905339788 ) ) ;
#31376=VECTOR ( 'NONE', #36132, 999.9999999999998863 ) ;
#31410=CARTESIAN_POINT ( 'NONE',  ( -16.09647726239903776, 23.36497036543017813, -3.956233406722669432 ) ) ;
#31418=CARTESIAN_POINT ( 'NONE',  ( -21.93567466420777379, 19.99370817364452790, -4.408991681665293427 ) ) ;
#31429=ORIENTED_EDGE ( 'NONE', *, *, #42479, .F. ) ;
#31476=CARTESIAN_POINT ( 'NONE',  ( -22.36868959911851462, 19.74370688441071309, 4.433756599430258127 ) ) ;
#31526=CARTESIAN_POINT ( 'NONE',  ( -20.66714045964574709, 20.62987310936011909, 4.333808234688889094 ) ) ;
#31532=SURFACE_STYLE_FILL_AREA ( #52529 ) ;
#31540=EDGE_CURVE ( 'NONE', #52053, #15174, #34874, .T. ) ;
#31565=EDGE_CURVE ( 'NONE', #15218, #17024, #56169, .T. ) ;
#31567=ORIENTED_EDGE ( 'NONE', *, *, #30287, .F. ) ;
#31575=CARTESIAN_POINT ( 'NONE',  ( -24.74852218546340410, 18.25476860917765620, -4.557895514311181451 ) ) ;
#31627=ORIENTED_EDGE ( 'NONE', *, *, #5695, .T. ) ;
#31658=CARTESIAN_POINT ( 'NONE',  ( -24.53375310857961367, 18.49370688441070953, 4.545578210335888159 ) ) ;
#31660=DIRECTION ( 'NONE',  ( -0.7886751345948130876, 0.2113248654051844977, -0.5773502691896263972 ) ) ;
#31663=FACE_OUTER_BOUND ( 'NONE', #3887, .T. ) ;
#31666=COLOUR_RGB ( '', 0.40784314, 0.44705882, 0.49803922) ;
#31681=CARTESIAN_POINT ( 'NONE',  ( -14.70243142924463875, 24.16982310246453380, -3.792938838976426918 ) ) ;
#31739=B_SPLINE_CURVE_WITH_KNOTS ( 'NONE', 3,
 ( #39196, #16490, #29586, #55682 ),
 .UNSPECIFIED., .F., .F.,
 ( 4, 4 ),
 ( 0.0002809688904423142679, 0.0003536739149152803505 ),
 .UNSPECIFIED. ) ;
#31746=CARTESIAN_POINT ( 'NONE',  ( -23.29661994227107868, 19.01267450544941084, 4.488313114961025363 ) ) ;
#31783=VERTEX_POINT ( 'NONE', #13505 ) ;
#31799=DIRECTION ( 'NONE',  ( -0.3583679495452925523, -0.9335804264972047406, -0.000000000000000000 ) ) ;
#31854=ORIENTED_EDGE ( 'NONE', *, *, #40489, .F. ) ;
#31858=CIRCLE ( 'NONE', #7361, 0.5000000000000004441 ) ;
#31892=PRODUCT ( 'Upper Lever Press Arm', 'Upper Lever Press Arm', '', ( #34319 ) ) ;
#31913=LINE ( 'NONE', #39878, #2193 ) ;
#31916=PLANE ( 'NONE',  #54161 ) ;
#31925=EDGE_CURVE ( 'NONE', #54860, #12684, #1509, .T. ) ;
#31940=AXIS2_PLACEMENT_3D ( 'NONE', #4537, #17900, #51941 ) ;
#31994=ORIENTED_EDGE ( 'NONE', *, *, #44141, .F. ) ;
#32007=CARTESIAN_POINT ( 'NONE',  ( -33.75052341732683914, 11.44035125802762032, 4.909800093382857611 ) ) ;
#32041=ORIENTED_EDGE ( 'NONE', *, *, #27857, .F. ) ;
#32120=ORIENTED_EDGE ( 'NONE', *, *, #31925, .T. ) ;
#32125=ORIENTED_EDGE ( 'NONE', *, *, #11093, .T. ) ;
#32140=CARTESIAN_POINT ( 'NONE',  ( -56.70083583094844926, 4.876814673940706335, 2.999999999999993339 ) ) ;
#32172=CARTESIAN_POINT ( 'NONE',  ( -24.96676581047183063, 18.24370688441070953, -4.657437592157546824 ) ) ;
#32181=ORIENTED_EDGE ( 'NONE', *, *, #19403, .T. ) ;
#32191=VERTEX_POINT ( 'NONE', #29349 ) ;
#32212=CARTESIAN_POINT ( 'NONE',  ( -24.56000334535257679, 18.39573966706334929, 4.548402587786432250 ) ) ;
#32230=VECTOR ( 'NONE', #6091, 1000.000000000000000 ) ;
#32245=CARTESIAN_POINT ( 'NONE',  ( -56.66762604419704985, 5.055998648713356580, 2.999999999999993339 ) ) ;
#32261=CARTESIAN_POINT ( 'NONE',  ( -29.08986725154028363, 15.86323315751366358, 4.728329674295676632 ) ) ;
#32274=CIRCLE ( 'NONE', #42225, 0.5000000000000004441 ) ;
#32393=EDGE_CURVE ( 'NONE', #24617, #27675, #48658, .T. ) ;
#32396=VECTOR ( 'NONE', #6376, 1000.000000000000000 ) ;
#32407=AXIS2_PLACEMENT_3D ( 'NONE', #13288, #3622, #8172 ) ;
#32418=CARTESIAN_POINT ( 'NONE',  ( -24.66083326546969801, 18.30078199617196688, -4.553899816365563957 ) ) ;
#32448=ORIENTED_EDGE ( 'NONE', *, *, #30287, .T. ) ;
#32522=CARTESIAN_POINT ( 'NONE',  ( -19.92277643783922869, 21.15585550648971491, -4.281362112901368810 ) ) ;
#32535=CARTESIAN_POINT ( 'NONE',  ( -29.16342252716179928, 15.82076599933325944, 4.730794752401083159 ) ) ;
#32547=PLANE ( 'NONE',  #1498 ) ;
#32556=CARTESIAN_POINT ( 'NONE',  ( -32.77407650832405750, 13.73615395135863970, -4.840648455043430332 ) ) ;
#32561=ORIENTED_EDGE ( 'NONE', *, *, #26676, .F. ) ;
#32566=CARTESIAN_POINT ( 'NONE',  ( -24.24106128977693331, 18.66269258478600079, -4.531817629136046577 ) ) ;
#32581=STYLED_ITEM ( 'NONE', ( #1405 ), #27288 ) ;
#32602=DIRECTION ( 'NONE',  ( 0.8660254037844380415, 0.5000000000000011102, 0.000000000000000000 ) ) ;
#32621=CARTESIAN_POINT ( 'NONE',  ( -11.13054826722768098, 24.50000000000005684, 3.000000000000000444 ) ) ;
#32628=CARTESIAN_POINT ( 'NONE',  ( -61.10213307005876260, 6.758246409053501047, 2.999999999999993339 ) ) ;
#32640=ORIENTED_EDGE ( 'NONE', *, *, #55662, .F. ) ;
#32694=CARTESIAN_POINT ( 'NONE',  ( -25.83906187201940341, 17.72030447104181050, 4.604772761472839981 ) ) ;
#32706=DIRECTION ( 'NONE',  ( 0.3583679495452925523, 0.9335804264972047406, 0.000000000000000000 ) ) ;
#32711=EDGE_LOOP ( 'NONE', ( #13857, #8940, #26000, #5382, #26299, #7222 ) ) ;
#32716=CARTESIAN_POINT ( 'NONE',  ( -19.42910703681909368, 21.15220053346460816, -4.255330291692488665 ) ) ;
#32726=LINE ( 'NONE', #50341, #44729 ) ;
#32736=VECTOR ( 'NONE', #18790, 1000.000000000000000 ) ;
#32751=EDGE_CURVE ( 'NONE', #11552, #26953, #19018, .T. ) ;
#32777=CARTESIAN_POINT ( 'NONE',  ( -11.36804826722768524, 24.91136206679766474, -3.000000000000000000 ) ) ;
#32800=CARTESIAN_POINT ( 'NONE',  ( -19.77061338776520216, 21.24370688441071664, -4.270683379717145733 ) ) ;
#32802=DIRECTION ( 'NONE',  ( 0.000000000000000000, -0.000000000000000000, -1.000000000000000000 ) ) ;
#32809=CARTESIAN_POINT ( 'NONE',  ( -29.09713277628012307, 15.85903840484930960, -4.728573048006373014 ) ) ;
#32828=B_SPLINE_CURVE_WITH_KNOTS ( 'NONE', 3,
 ( #23662, #44409, #39877, #18580 ),
 .UNSPECIFIED., .F., .F.,
 ( 4, 4 ),
 ( 0.3889078242859423939, 0.4131271774438034505 ),
 .UNSPECIFIED. ) ;
#32877=CARTESIAN_POINT ( 'NONE',  ( -11.91804826722769306, 25.86399001096056338, 4.999999999999888978 ) ) ;
#32936=ORIENTED_EDGE ( 'NONE', *, *, #15013, .F. ) ;
#32940=CARTESIAN_POINT ( 'NONE',  ( -50.99228148001754590, 2.341865487272627000, -5.000000000000000000 ) ) ;
#32976=CARTESIAN_POINT ( 'NONE',  ( -50.02554558092695913, 3.776013638374817294, 5.000000000000000000 ) ) ;
#32982=EDGE_LOOP ( 'NONE', ( #8563, #2485, #34800, #48358 ) ) ;
#32988=ORIENTED_EDGE ( 'NONE', *, *, #32751, .F. ) ;
#33041=CARTESIAN_POINT ( 'NONE',  ( -62.23823698199103660, 6.658783344088820222, 3.000000000000000000 ) ) ;
#33074=VECTOR ( 'NONE', #16005, 1000.000000000000114 ) ;
#33104=CIRCLE ( 'NONE', #12263, 0.5000000000000004441 ) ;
#33111=EDGE_CURVE ( 'NONE', #50858, #21631, #18112, .T. ) ;
#33149=ORIENTED_EDGE ( 'NONE', *, *, #18824, .T. ) ;
#33196=VECTOR ( 'NONE', #9426, 1000.000000000000114 ) ;
#33209=CARTESIAN_POINT ( 'NONE',  ( -23.29661890453421691, 19.01267837833611551, -4.488312987714206059 ) ) ;
#33272=EDGE_CURVE ( 'NONE', #5918, #11612, #16031, .T. ) ;
#33292=ORIENTED_EDGE ( 'NONE', *, *, #31925, .F. ) ;
#33304=B_SPLINE_CURVE_WITH_KNOTS ( 'NONE', 3,
 ( #20843, #46690, #17723, #17159 ),
 .UNSPECIFIED., .F., .F.,
 ( 4, 4 ),
 ( 0.000000000000000000, 0.0003538274413750240122 ),
 .UNSPECIFIED. ) ;
#33338=EDGE_LOOP ( 'NONE', ( #4791, #51722, #7177, #28517 ) ) ;
#33348=ORIENTED_EDGE ( 'NONE', *, *, #12341, .T. ) ;
#33392=DIRECTION ( 'NONE',  ( -0.7886751345948130876, 0.2113248654051844977, 0.5773502691896263972 ) ) ;
#33400=VERTEX_POINT ( 'NONE', #39579 ) ;
#33406=EDGE_CURVE ( 'NONE', #18987, #36742, #36648, .T. ) ;
#33412=CARTESIAN_POINT ( 'NONE',  ( -20.59425094460877403, 20.76817951925234951, 4.326372769521754869 ) ) ;
#33476=CARTESIAN_POINT ( 'NONE',  ( -21.93567689722629765, 19.99370688441071309, 4.657440554554202805 ) ) ;
#33502=EDGE_CURVE ( 'NONE', #17567, #45180, #29123, .T. ) ;
#33541=CARTESIAN_POINT ( 'NONE',  ( -25.84533253705052047, 17.69690203054840794, 4.605409525904272883 ) ) ;
#33579=ORIENTED_EDGE ( 'NONE', *, *, #41766, .T. ) ;
#33593=EDGE_CURVE ( 'NONE', #14093, #4092, #11412, .T. ) ;
#33597=EDGE_CURVE ( 'NONE', #48717, #460, #46902, .T. ) ;
#33606=CARTESIAN_POINT ( 'NONE',  ( -61.74810725808001877, 6.470640170577545369, 2.999999999999993339 ) ) ;
#33655=EDGE_CURVE ( 'NONE', #15174, #22670, #16221, .T. ) ;
#33669=CARTESIAN_POINT ( 'NONE',  ( -20.43612818448172419, 20.85947173737672955, 4.315991441970404630 ) ) ;
#33679=B_SPLINE_CURVE_WITH_KNOTS ( 'NONE', 3,
 ( #55315, #16410, #30051, #47085, #47356, #33734, #52195, #8466, #4496, #20949, #4233, #21803, #12161, #17003, #42550, #29496, #46816, #38862, #16707, #34037, #25795, #14428, #18961, #1634, #36278, #39421, #39710, #32007, #23227, #5604 ),
 .UNSPECIFIED., .F., .F.,
 ( 4, 1, 1, 1, 1, 1, 1, 1, 1, 1, 1, 2, 2, 1, 1, 1, 1, 1, 1, 1, 1, 2, 2, 4 ),
 ( 0.000000000000000000, 0.1249999999997620792, 0.1874999999996430633, 0.2187499999995836386, 0.2343749999995539124, 0.2421874999995391464, 0.2460937499995317357, 0.2480468749995280442, 0.2490234374995262401, 0.2495117187495253241, 0.2497558593745249633, 0.2498779296870247690, 0.2499999999995246025, 0.3749999999996284084, 0.4374999999996804223, 0.4687499999997064570, 0.4843749999997194466, 0.4921874999997258859, 0.4960937499997292166, 0.4980468749997308819, 0.4990234374997316591, 0.4995117187497319922, 0.4999999999997323252, 1.000000000000000000 ),
 .UNSPECIFIED. ) ;
#33700=ORIENTED_EDGE ( 'NONE', *, *, #37372, .T. ) ;
#33708=CIRCLE ( 'NONE', #23746, 2.000000000000002220 ) ;
#33720=FACE_OUTER_BOUND ( 'NONE', #20007, .T. ) ;
#33734=CARTESIAN_POINT ( 'NONE',  ( -18.47181751008412220, 20.26151622644335148, 4.232279298899151776 ) ) ;
#33746=ORIENTED_EDGE ( 'NONE', *, *, #39119, .F. ) ;
#33767=ADVANCED_FACE ( 'NONE', ( #21031 ), #51698, .F. ) ;
#33794=CARTESIAN_POINT ( 'NONE',  ( -46.52156441860571334, 5.799038105676371124, -5.000000000000000000 ) ) ;
#33811=EDGE_CURVE ( 'NONE', #48202, #16580, #7915, .T. ) ;
#33823=DIRECTION ( 'NONE',  ( 0.2113248654051873565, 0.7886751345948121994, -0.5773502691896263972 ) ) ;
#33840=ORIENTED_EDGE ( 'NONE', *, *, #14552, .F. ) ;
#33847=DIRECTION ( 'NONE',  ( 0.3583679495452925523, 0.9335804264972047406, 0.000000000000000000 ) ) ;
#33849=DIRECTION ( 'NONE',  ( -0.2588190451025176864, -0.9659258262890692004, 0.000000000000000000 ) ) ;
#33854=LINE ( 'NONE', #24230, #17756 ) ;
#33884=MECHANICAL_DESIGN_GEOMETRIC_PRESENTATION_REPRESENTATION('',(#19357),#39317);
#33965=CARTESIAN_POINT ( 'NONE',  ( -19.77061338776520216, 21.24370688441071664, 4.270755533188014930 ) ) ;
#33979=ORIENTED_EDGE ( 'NONE', *, *, #45565, .T. ) ;
#34037=CARTESIAN_POINT ( 'NONE',  ( -27.65699453300243249, 14.95845179970709182, 4.704869143278580523 ) ) ;
#34040=AXIS2_PLACEMENT_3D ( 'NONE', #8965, #13220, #22305 ) ;
#34066=CARTESIAN_POINT ( 'NONE',  ( -23.32622135384906770, 18.90220053346460105, 4.407440554554201917 ) ) ;
#34077=VECTOR ( 'NONE', #42455, 1000.000000000000000 ) ;
#34084=ADVANCED_FACE ( 'NONE', ( #25774 ), #39403, .F. ) ;
#34131=AXIS2_PLACEMENT_3D ( 'NONE', #47985, #48837, #9084 ) ;
#34162=ORIENTED_EDGE ( 'NONE', *, *, #14291, .F. ) ;
#34212=CARTESIAN_POINT ( 'NONE',  ( -50.02554558092695913, 3.776013638374817294, 5.000000000000000000 ) ) ;
#34258=DIRECTION ( 'NONE',  ( 1.000000000000000000, 0.000000000000000000, 0.000000000000000000 ) ) ;
#34268=DIRECTION ( 'NONE',  ( -0.7886751345948130876, 0.2113248654051844977, -0.5773502691896263972 ) ) ;
#34319=PRODUCT_CONTEXT ( 'NONE', #13390, 'mechanical' ) ;
#34399=ORIENTED_EDGE ( 'NONE', *, *, #8617, .T. ) ;
#34412=CARTESIAN_POINT ( 'NONE',  ( -64.10539783498545319, 7.375519243179410545, -3.000000000000000000 ) ) ;
#34421=ORIENTED_EDGE ( 'NONE', *, *, #13492, .F. ) ;
#34425=CARTESIAN_POINT ( 'NONE',  ( -56.48844206942440138, 5.522788861961955398, 2.999999999999993339 ) ) ;
#34450=VERTEX_POINT ( 'NONE', #8504 ) ;
#34457=CARTESIAN_POINT ( 'NONE',  ( -24.57312852195785524, 18.34675584111407787, 4.549864924635812713 ) ) ;
#34479=DIRECTION ( 'NONE',  ( 0.3535533905932738974, -0.6123724356957929160, 0.7071067811865487940 ) ) ;
#34493=EDGE_CURVE ( 'NONE', #45180, #18779, #23257, .T. ) ;
#34519=CARTESIAN_POINT ( 'NONE',  ( -22.03895693409927858, 19.66185913055325685, -4.421689025564675468 ) ) ;
#34559=CYLINDRICAL_SURFACE ( 'NONE', #32407, 0.5000000000000004441 ) ;
#34575=CARTESIAN_POINT ( 'NONE',  ( -50.02554558092695913, 3.776013638374817294, 5.000000000000000000 ) ) ;
#34633=LINE ( 'NONE', #43449, #49729 ) ;
#34638=CARTESIAN_POINT ( 'NONE',  ( 0.000000000000000000, 0.000000000000000000, 0.000000000000000000 ) ) ;
#34711=VERTEX_POINT ( 'NONE', #14656 ) ;
#34752=VECTOR ( 'NONE', #48748, 1000.000000000000114 ) ;
#34757=CARTESIAN_POINT ( 'NONE',  ( -23.66772770479517618, 18.99370688441070953, 4.503109509781816122 ) ) ;
#34760=CARTESIAN_POINT ( 'NONE',  ( -11.13054826722768098, 24.50000000000005684, -3.000000000000000000 ) ) ;
#34800=ORIENTED_EDGE ( 'NONE', *, *, #20617, .F. ) ;
#34812=VERTEX_POINT ( 'NONE', #32800 ) ;
#34818=ORIENTED_EDGE ( 'NONE', *, *, #36328, .F. ) ;
#34832=AXIS2_PLACEMENT_3D ( 'NONE', #49624, #36847, #53856 ) ;
#34874=LINE ( 'NONE', #34575, #48611 ) ;
#34945=CARTESIAN_POINT ( 'NONE',  ( -21.99342909152279191, 19.77817276104758193, -4.416855321001344592 ) ) ;
#35015=EDGE_CURVE ( 'NONE', #24159, #41243, #47277, .T. ) ;
#35021=CARTESIAN_POINT ( 'NONE',  ( -50.99228148001754590, 2.341865487272625668, 5.000000000000000000 ) ) ;
#35044=B_SPLINE_CURVE_WITH_KNOTS ( 'NONE', 3,
 ( #26021, #12661, #4149, #43335 ),
 .UNSPECIFIED., .F., .F.,
 ( 4, 4 ),
 ( 0.6614527403836476527, 0.6877732163401213406 ),
 .UNSPECIFIED. ) ;
#35045=AXIS2_PLACEMENT_3D ( 'NONE', #19472, #36815, #9860 ) ;
#35192=ORIENTED_EDGE ( 'NONE', *, *, #38990, .F. ) ;
#35204=DIRECTION ( 'NONE',  ( -1.000000000000000000, 0.000000000000000000, 0.000000000000000000 ) ) ;
#35213=DIRECTION ( 'NONE',  ( -1.000000000000000000, 0.000000000000000000, 0.000000000000000000 ) ) ;
#35247=EDGE_CURVE ( 'NONE', #54087, #19901, #32726, .T. ) ;
#35257=ORIENTED_EDGE ( 'NONE', *, *, #5710, .T. ) ;
#35286=DIRECTION ( 'NONE',  ( 0.000000000000000000, 0.000000000000000000, -1.000000000000000000 ) ) ;
#35305=CARTESIAN_POINT ( 'NONE',  ( -24.83619032682412353, 18.20871928901600256, 4.561852666301203563 ) ) ;
#35307=CARTESIAN_POINT ( 'NONE',  ( -11.88054826722768276, 25.79903810567671130, -3.000000000000000000 ) ) ;
#35338=DIRECTION ( 'NONE',  ( 0.2113248654051873565, 0.7886751345948123104, 0.5773502691896265082 ) ) ;
#35359=DIRECTION ( 'NONE',  ( 1.000000000000000000, 0.000000000000000000, -8.673617379884027583E-16 ) ) ;
#35423=CARTESIAN_POINT ( 'NONE',  ( -28.66953870280127248, 14.37385915070733944, -4.739290323461024634 ) ) ;
#35442=ORIENTED_EDGE ( 'NONE', *, *, #50895, .T. ) ;
#35461=ADVANCED_FACE ( 'NONE', ( #17109 ), #51729, .F. ) ;
#35477=DIRECTION ( 'NONE',  ( 1.000000000000000000, 0.000000000000000000, 0.000000000000000000 ) ) ;
#35494=EDGE_LOOP ( 'NONE', ( #35951, #8928, #4529, #38037 ) ) ;
#35546=CARTESIAN_POINT ( 'NONE',  ( -27.33717112119440174, 16.68270265044663603, 4.490773887887534954 ) ) ;
#35562=DIRECTION ( 'NONE',  ( -1.000000000000000000, 0.000000000000000000, 0.000000000000000000 ) ) ;
#35581=DIRECTION ( 'NONE',  ( 0.2113248654051873565, 0.7886751345948121994, -0.5773502691896263972 ) ) ;
#35610=SURFACE_STYLE_FILL_AREA ( #18278 ) ;
#35614=ORIENTED_EDGE ( 'NONE', *, *, #518, .T. ) ;
#35635=LINE ( 'NONE', #36761, #32396 ) ;
#35646=B_SPLINE_CURVE_WITH_KNOTS ( 'NONE', 3,
 ( #33794, #12220, #27235, #30393 ),
 .UNSPECIFIED., .F., .F.,
 ( 4, 4 ),
 ( 0.000000000000000000, 1.000000000000000000 ),
 .UNSPECIFIED. ) ;
#35656=ORIENTED_EDGE ( 'NONE', *, *, #44650, .F. ) ;
#35712=CARTESIAN_POINT ( 'NONE',  ( -19.69488366597744289, 19.55537865210161996, -4.316569728936750394 ) ) ;
#35729=CARTESIAN_POINT ( 'NONE',  ( -24.62525945952572215, 18.15220053346460105, -4.407437592157546824 ) ) ;
#35764=CARTESIAN_POINT ( 'NONE',  ( -19.77061338776520216, 21.24370688441071664, -4.657437592157546824 ) ) ;
#35794=AXIS2_PLACEMENT_3D ( 'NONE', #43636, #48171, #47922 ) ;
#35895=DIRECTION ( 'NONE',  ( 0.000000000000000000, 0.000000000000000000, 1.000000000000000000 ) ) ;
#35896=VERTEX_POINT ( 'NONE', #28018 ) ;
#35949=VECTOR ( 'NONE', #35581, 1000.000000000000114 ) ;
#35951=ORIENTED_EDGE ( 'NONE', *, *, #31565, .T. ) ;
#35993=VERTEX_POINT ( 'NONE', #20867 ) ;
#36045=AXIS2_PLACEMENT_3D ( 'NONE', #34212, #39282, #8927 ) ;
#36071=DIRECTION ( 'NONE',  ( 1.000000000000000000, 0.000000000000000000, 0.000000000000000000 ) ) ;
#36132=DIRECTION ( 'NONE',  ( 0.9335804264972041855, -0.3583679495452943287, 0.000000000000000000 ) ) ;
#36169=ORIENTED_EDGE ( 'NONE', *, *, #46464, .F. ) ;
#36223=CARTESIAN_POINT ( 'NONE',  ( -20.51047058032500559, 20.81655013512439822, -4.320899323597838126 ) ) ;
#36232=ADVANCED_FACE ( 'NONE', ( #51261 ), #47008, .F. ) ;
#36278=CARTESIAN_POINT ( 'NONE',  ( -28.34606951297313060, 14.56061417452916729, 4.728537094605865576 ) ) ;
#36292=LINE ( 'NONE', #5927, #15824 ) ;
#36328=EDGE_CURVE ( 'NONE', #5918, #42224, #31913, .T. ) ;
#36454=DIRECTION ( 'NONE',  ( -0.3583679495452941621, -0.9335804264972042965, 0.000000000000000000 ) ) ;
#36476=ORIENTED_EDGE ( 'NONE', *, *, #9773, .F. ) ;
#36482=CARTESIAN_POINT ( 'NONE',  ( -20.63663870328428374, 20.74370693537071020, -4.329125112780540796 ) ) ;
#36503=EDGE_CURVE ( 'NONE', #48024, #44358, #56027, .T. ) ;
#36505=CARTESIAN_POINT ( 'NONE',  ( -26.83479864408084126, 17.16519762507144975, 4.645878820492973738 ) ) ;
#36576=ORIENTED_EDGE ( 'NONE', *, *, #29222, .T. ) ;
#36632=ORIENTED_EDGE ( 'NONE', *, *, #7444, .F. ) ;
#36642=DIRECTION ( 'NONE',  ( 0.000000000000000000, 0.000000000000000000, 1.000000000000000000 ) ) ;
#36648=B_SPLINE_CURVE_WITH_KNOTS ( 'NONE', 3,
 ( #26779, #13452, #9171, #35307 ),
 .UNSPECIFIED., .F., .F.,
 ( 4, 4 ),
 ( 0.000000000000000000, 1.000000000000000000 ),
 .UNSPECIFIED. ) ;
#36701=CARTESIAN_POINT ( 'NONE',  ( -19.33760068587298164, 21.49370688441072019, 4.239878526350478793 ) ) ;
#36714=ORIENTED_EDGE ( 'NONE', *, *, #26825, .T. ) ;
#36725=CARTESIAN_POINT ( 'NONE',  ( -27.56484202182514665, 16.74370688441070953, -4.657437592157546824 ) ) ;
#36742=VERTEX_POINT ( 'NONE', #7388 ) ;
#36745=LINE ( 'NONE', #22071, #14921 ) ;
#36751=LINE ( 'NONE', #14347, #54838 ) ;
#36761=CARTESIAN_POINT ( 'NONE',  ( -50.99228148001754590, 2.341865487272625668, 5.000000000000000000 ) ) ;
#36815=DIRECTION ( 'NONE',  ( 0.3535533905932752297, -0.6123724356957952475, -0.7071067811865462405 ) ) ;
#36847=DIRECTION ( 'NONE',  ( 0.000000000000000000, 0.000000000000000000, -1.000000000000000000 ) ) ;
#36867=AXIS2_PLACEMENT_3D ( 'NONE', #5275, #974, #34258 ) ;
#36898=CARTESIAN_POINT ( 'NONE',  ( -27.13182931993292257, 16.99370688441070953, -4.657437592157546824 ) ) ;
#36925=VERTEX_POINT ( 'NONE', #56217 ) ;
#36974=EDGE_CURVE ( 'NONE', #42260, #17024, #17656, .T. ) ;
#37003=CARTESIAN_POINT ( 'NONE',  ( -46.52156441860518754, 5.799038105676674881, 5.000000000000000000 ) ) ;
#37008=CARTESIAN_POINT ( 'NONE',  ( -24.62525945952572215, 18.15220053346459750, 4.407440554554201917 ) ) ;
#37009=EDGE_CURVE ( 'NONE', #11612, #48717, #33104, .T. ) ;
#37023=ORIENTED_EDGE ( 'NONE', *, *, #12836, .F. ) ;
#37039=EDGE_CURVE ( 'NONE', #43487, #27671, #46342, .T. ) ;
#37061=CARTESIAN_POINT ( 'NONE',  ( -11.09304826722767956, 24.43504809471621542, -3.000000000000000000 ) ) ;
#37067=VERTEX_POINT ( 'NONE', #13366 ) ;
#37071=CARTESIAN_POINT ( 'NONE',  ( -24.24107053542677548, 18.66268724680757884, 4.531816173043640816 ) ) ;
#37075=CARTESIAN_POINT ( 'NONE',  ( -27.13182803479460858, 16.99370762638562127, 4.657392947539034544 ) ) ;
#37080=ORIENTED_EDGE ( 'NONE', *, *, #33655, .T. ) ;
#37083=DIRECTION ( 'NONE',  ( -0.7886751345948130876, 0.2113248654051844977, 0.5773502691896263972 ) ) ;
#37107=FACE_OUTER_BOUND ( 'NONE', #6683, .T. ) ;
#37133=ORIENTED_EDGE ( 'NONE', *, *, #2855, .T. ) ;
#37153=DIRECTION ( 'NONE',  ( 0.9659258262890682012, -0.2588190451025213501, 0.000000000000000000 ) ) ;
#37155=CARTESIAN_POINT ( 'NONE',  ( -27.13182931993292257, 16.99370688441070953, 4.657440554554202805 ) ) ;
#37251=EDGE_CURVE ( 'NONE', #15218, #54860, #54853, .T. ) ;
#37332=ORIENTED_EDGE ( 'NONE', *, *, #27857, .T. ) ;
#37372=EDGE_CURVE ( 'NONE', #49975, #9690, #17926, .T. ) ;
#37432=EDGE_CURVE ( 'NONE', #607, #27671, #28782, .T. ) ;
#37557=( LENGTH_UNIT ( ) NAMED_UNIT ( * ) SI_UNIT ( .MILLI., .METRE. ) );
#37558=DIRECTION ( 'NONE',  ( -0.2588190451025176864, -0.9659258262890692004, 0.000000000000000000 ) ) ;
#37638=ORIENTED_EDGE ( 'NONE', *, *, #45571, .F. ) ;
#37647=CARTESIAN_POINT ( 'NONE',  ( -42.47825799898742360, 8.133442155459132294, -4.990245731342549007 ) ) ;
#37705=VERTEX_POINT ( 'NONE', #47925 ) ;
#37733=AXIS2_PLACEMENT_3D ( 'NONE', #38335, #3981, #55659 ) ;
#37785=CARTESIAN_POINT ( 'NONE',  ( -26.11787696043622375, 17.53257130528676910, 4.617134652480109125 ) ) ;
#37824=AXIS2_PLACEMENT_3D ( 'NONE', #7189, #37558, #21072 ) ;
#37843=ORIENTED_EDGE ( 'NONE', *, *, #48391, .T. ) ;
#37861=( NAMED_UNIT ( * ) PLANE_ANGLE_UNIT ( ) SI_UNIT ( $, .RADIAN. ) );
#37878=ORIENTED_EDGE ( 'NONE', *, *, #19434, .F. ) ;
#38015=DIRECTION ( 'NONE',  ( 0.3535533905932752297, -0.6123724356957952475, 0.7071067811865462405 ) ) ;
#38037=ORIENTED_EDGE ( 'NONE', *, *, #12987, .T. ) ;
#38159=FACE_OUTER_BOUND ( 'NONE', #33338, .T. ) ;
#38171=CARTESIAN_POINT ( 'NONE',  ( -12.33635297242189921, 23.80382832886605726, -3.523096027145014464 ) ) ;
#38176=ORIENTED_EDGE ( 'NONE', *, *, #35015, .T. ) ;
#38282=EDGE_LOOP ( 'NONE', ( #8564, #32448, #52280 ) ) ;
#38323=DIRECTION ( 'NONE',  ( 1.000000000000000000, 0.000000000000000000, 0.000000000000000000 ) ) ;
#38335=CARTESIAN_POINT ( 'NONE',  ( -61.56892328330737030, 6.937430383826147740, 2.999999999999993339 ) ) ;
#38339=AXIS2_PLACEMENT_3D ( 'NONE', #54359, #2410, #50089 ) ;
#38351=EDGE_CURVE ( 'NONE', #26953, #12681, #21397, .T. ) ;
#38353=VERTEX_POINT ( 'NONE', #6116 ) ;
#38360=DIRECTION ( 'NONE',  ( -0.2588190451025212946, -0.9659258262890680902, 0.000000000000000000 ) ) ;
#38362=ORIENTED_EDGE ( 'NONE', *, *, #455, .F. ) ;
#38438=CARTESIAN_POINT ( 'NONE',  ( -63.00984630926864583, 1.788483511016180305, -3.000000000000007105 ) ) ;
#38450=AXIS2_PLACEMENT_3D ( 'NONE', #18091, #43102, #21533 ) ;
#38458=CARTESIAN_POINT ( 'NONE',  ( -12.31198489147366715, 23.81789724696114519, -3.517870358740663672 ) ) ;
#38572=ORIENTED_EDGE ( 'NONE', *, *, #17293, .F. ) ;
#38622=AXIS2_PLACEMENT_3D ( 'NONE', #15033, #49677, #49092 ) ;
#38679=AXIS2_PLACEMENT_3D ( 'NONE', #10948, #46712, #25154 ) ;
#38692=DIRECTION ( 'NONE',  ( -0.9335804264972049626, 0.3583679495452921082, 0.000000000000000000 ) ) ;
#38713=VECTOR ( 'NONE', #49825, 1000.000000000000000 ) ;
#38714=DIRECTION ( 'NONE',  ( 0.2113248654051873565, 0.7886751345948121994, -0.5773502691896263972 ) ) ;
#38767=CARTESIAN_POINT ( 'NONE',  ( -11.13054826722768098, 24.50000000000005684, 5.000000000000000000 ) ) ;
#38807=CARTESIAN_POINT ( 'NONE',  ( -25.83278826518980154, 17.74370858705499288, -4.604226652742015702 ) ) ;
#38814=LINE ( 'NONE', #16647, #52170 ) ;
#38832=EDGE_CURVE ( 'NONE', #37067, #11552, #1107, .T. ) ;
#38862=CARTESIAN_POINT ( 'NONE',  ( -25.57735469142784979, 16.15913242205765599, 4.626755875664946949 ) ) ;
#38872=ORIENTED_EDGE ( 'NONE', *, *, #42479, .T. ) ;
#38882=EDGE_CURVE ( 'NONE', #24617, #30957, #21861, .T. ) ;
#38990=EDGE_CURVE ( 'NONE', #10403, #53934, #24420, .T. ) ;
#39024=CARTESIAN_POINT ( 'NONE',  ( -13.23914656339586315, 23.28260020609454983, -3.687136209236635764 ) ) ;
#39036=ORIENTED_EDGE ( 'NONE', *, *, #44338, .F. ) ;
#39047=ORIENTED_EDGE ( 'NONE', *, *, #12987, .F. ) ;
#39063=B_SPLINE_CURVE_WITH_KNOTS ( 'NONE', 3,
 ( #3675, #20446, #37785, #11908 ),
 .UNSPECIFIED., .F., .F.,
 ( 4, 4 ),
 ( 5.447042101129314832E-05, 0.0005066785541756341910 ),
 .UNSPECIFIED. ) ;
#39092=ORIENTED_EDGE ( 'NONE', *, *, #5926, .T. ) ;
#39117=CARTESIAN_POINT ( 'NONE',  ( -33.30197399026911853, 11.69932139048425235, -4.869895353451894060 ) ) ;
#39119=EDGE_CURVE ( 'NONE', #48024, #48202, #12160, .T. ) ;
#39194=EDGE_LOOP ( 'NONE', ( #31854, #41938, #23041 ) ) ;
#39196=CARTESIAN_POINT ( 'NONE',  ( -25.85160216376510434, 17.67350346510513148, -4.606045122360801436 ) ) ;
#39226=ORIENTED_EDGE ( 'NONE', *, *, #38990, .T. ) ;
#39250=PLANE ( 'NONE',  #7058 ) ;
#39254=CARTESIAN_POINT ( 'NONE',  ( -25.97317167826694728, 17.60920382705421261, -4.611144759605506849 ) ) ;
#39282=DIRECTION ( 'NONE',  ( 0.5000000000000011102, -0.8660254037844380415, 0.000000000000000000 ) ) ;
#39303=ORIENTED_EDGE ( 'NONE', *, *, #49130, .F. ) ;
#39317=( GEOMETRIC_REPRESENTATION_CONTEXT ( 3 ) GLOBAL_UNCERTAINTY_ASSIGNED_CONTEXT ( ( #21150 ) ) GLOBAL_UNIT_ASSIGNED_CONTEXT ( ( #37557, #37861, #50039 ) ) REPRESENTATION_CONTEXT ( 'NONE', 'WORKASPACE' ) );
#39331=PLANE ( 'NONE',  #43805 ) ;
#39337=DIRECTION ( 'NONE',  ( 1.007958083594381669E-15, -3.869188571150966625E-16, 1.000000000000000000 ) ) ;
#39350=CARTESIAN_POINT ( 'NONE',  ( -15.89757661009962320, 23.47980571057722443, -3.935101339868287251 ) ) ;
#39403=PLANE ( 'NONE',  #38450 ) ;
#39413=CARTESIAN_POINT ( 'NONE',  ( -19.74387268839167575, 19.52709482682342923, -4.319799108532053289 ) ) ;
#39421=CARTESIAN_POINT ( 'NONE',  ( -28.35892388567684108, 14.55319269898841661, 4.728968845017322842 ) ) ;
#39422=CARTESIAN_POINT ( 'NONE',  ( -22.04727804374295275, 19.65758491770980143, 4.422150965879553475 ) ) ;
#39434=CIRCLE ( 'NONE', #29457, 0.5000000000000004441 ) ;
#39502=CYLINDRICAL_SURFACE ( 'NONE', #22282, 0.5000000000000004441 ) ;
#39541=DIRECTION ( 'NONE',  ( 0.000000000000000000, -0.000000000000000000, -1.000000000000000000 ) ) ;
#39572=VECTOR ( 'NONE', #18866, 1000.000000000000000 ) ;
#39579=CARTESIAN_POINT ( 'NONE',  ( -62.23823698199102950, 6.658783344088819334, -5.000000000000000000 ) ) ;
#39642=AXIS2_PLACEMENT_3D ( 'NONE', #24765, #33849, #16245 ) ;
#39670=ORIENTED_EDGE ( 'NONE', *, *, #4543, .T. ) ;
#39703=CARTESIAN_POINT ( 'NONE',  ( -26.72368083891871748, 15.49730071222468553, -4.674120403987057415 ) ) ;
#39710=CARTESIAN_POINT ( 'NONE',  ( -28.36653009681956661, 14.54880125093765386, 4.729224108455964526 ) ) ;
#39714=EDGE_CURVE ( 'NONE', #35993, #40047, #9565, .T. ) ;
#39727=VERTEX_POINT ( 'NONE', #42047 ) ;
#39731=DIRECTION ( 'NONE',  ( -0.8660254037844379305, -0.5000000000000011102, 0.000000000000000000 ) ) ;
#39738=CARTESIAN_POINT ( 'NONE',  ( -56.70083583094844926, 4.876814673940706335, -3.000000000000007105 ) ) ;
#39800=VERTEX_POINT ( 'NONE', #25568 ) ;
#39838=CARTESIAN_POINT ( 'NONE',  ( -23.52058925276516632, 18.95428125501370076, -4.498258577543088776 ) ) ;
#39852=EDGE_LOOP ( 'NONE', ( #53952, #35656, #48512, #50319, #10288, #51345 ) ) ;
#39877=CARTESIAN_POINT ( 'NONE',  ( -25.54040953336767927, 17.91251352657781482, -4.591766625787645495 ) ) ;
#39878=CARTESIAN_POINT ( 'NONE',  ( -50.99228148001754590, 2.341865487272625668, -3.000000000000007105 ) ) ;
#39905=CARTESIAN_POINT ( 'NONE',  ( -14.04345045867546915, 24.55028594321348123, -3.695677582892548774 ) ) ;
#39957=CARTESIAN_POINT ( 'NONE',  ( -29.57595708578221050, 13.85053825329486976, -4.768235699741624423 ) ) ;
#39990=ORIENTED_EDGE ( 'NONE', *, *, #16361, .T. ) ;
#40027=B_SPLINE_CURVE_WITH_KNOTS ( 'NONE', 3,
 ( #31476, #1050, #9299, #39422 ),
 .UNSPECIFIED., .F., .F.,
 ( 4, 4 ),
 ( 0.000000000000000000, 0.0003329496823836150814 ),
 .UNSPECIFIED. ) ;
#40047=VERTEX_POINT ( 'NONE', #53391 ) ;
#40055=ORIENTED_EDGE ( 'NONE', *, *, #36503, .F. ) ;
#40088=FACE_OUTER_BOUND ( 'NONE', #26878, .T. ) ;
#40126=ORIENTED_EDGE ( 'NONE', *, *, #33406, .T. ) ;
#40153=FACE_OUTER_BOUND ( 'NONE', #9261, .T. ) ;
#40160=FACE_OUTER_BOUND ( 'NONE', #24390, .T. ) ;
#40205=DIRECTION ( 'NONE',  ( -0.000000000000000000, -0.000000000000000000, 1.000000000000000000 ) ) ;
#40259=CARTESIAN_POINT ( 'NONE',  ( -23.23471500290295921, 19.24370688441070953, 4.480778704491060971 ) ) ;
#40308=FACE_OUTER_BOUND ( 'NONE', #21876, .T. ) ;
#40326=PLANE ( 'NONE',  #13287 ) ;
#40360=LINE ( 'NONE', #14517, #53101 ) ;
#40378=FACE_OUTER_BOUND ( 'NONE', #29283, .T. ) ;
#40396=VERTEX_POINT ( 'NONE', #27471 ) ;
#40448=LINE ( 'NONE', #6101, #39572 ) ;
#40478=ORIENTED_EDGE ( 'NONE', *, *, #28275, .T. ) ;
#40489=EDGE_CURVE ( 'NONE', #37705, #51242, #5001, .T. ) ;
#40506=ORIENTED_EDGE ( 'NONE', *, *, #38832, .T. ) ;
#40511=ORIENTED_EDGE ( 'NONE', *, *, #4499, .F. ) ;
#40512=LINE ( 'NONE', #23462, #5730 ) ;
#40574=B_SPLINE_CURVE_WITH_KNOTS ( 'NONE', 3,
 ( #41206, #19637, #49982, #11092 ),
 .UNSPECIFIED., .F., .F.,
 ( 4, 4 ),
 ( 0.000000000000000000, 0.0002286084161106520290 ),
 .UNSPECIFIED. ) ;
#40593=CARTESIAN_POINT ( 'NONE',  ( -11.91804826722769128, 25.86399001096056338, 3.000000000000000000 ) ) ;
#40655=DIRECTION ( 'NONE',  ( 0.8660254037844380415, 0.5000000000000011102, 0.000000000000000000 ) ) ;
#40703=ORIENTED_EDGE ( 'NONE', *, *, #50425, .F. ) ;
#40704=VERTEX_POINT ( 'NONE', #38807 ) ;
#40705=DIRECTION ( 'NONE',  ( 1.000000000000000000, -3.469446951953611033E-15, 0.000000000000000000 ) ) ;
#40718=CARTESIAN_POINT ( 'NONE',  ( -27.13182931993292257, 16.99370688441070953, 4.657440554554202805 ) ) ;
#40738=CARTESIAN_POINT ( 'NONE',  ( -20.84197899872283699, 20.43270222331197061, 4.347644189603123266 ) ) ;
#40740=( GEOMETRIC_REPRESENTATION_CONTEXT ( 3 ) GLOBAL_UNCERTAINTY_ASSIGNED_CONTEXT ( ( #24562 ) ) GLOBAL_UNIT_ASSIGNED_CONTEXT ( ( #48842, #582, #5663 ) ) REPRESENTATION_CONTEXT ( 'NONE', 'WORKASPACE' ) );
#40796=CARTESIAN_POINT ( 'NONE',  ( -37.76980095258905124, 10.85187109866503263, -4.935120467404106925 ) ) ;
#40814=DIRECTION ( 'NONE',  ( 0.3583679495452941066, 0.9335804264972041855, -0.000000000000000000 ) ) ;
#40835=DIRECTION ( 'NONE',  ( 0.000000000000000000, 0.000000000000000000, 1.000000000000000000 ) ) ;
#40859=DIRECTION ( 'NONE',  ( 0.000000000000000000, 0.000000000000000000, 1.000000000000000000 ) ) ;
#40870=AXIS2_PLACEMENT_3D ( 'NONE', #17364, #39541, #17108 ) ;
#40961=PRODUCT_DEFINITION_SHAPE ( 'NONE', 'NONE',  #18048 ) ;
#40970=CARTESIAN_POINT ( 'NONE',  ( -61.56892328330737740, 6.937430383826150404, -3.000000000000006661 ) ) ;
#41016=CARTESIAN_POINT ( 'NONE',  ( -50.02554558092695913, 3.776013638374815962, 5.000000000000000000 ) ) ;
#41051=ORIENTED_EDGE ( 'NONE', *, *, #45175, .F. ) ;
#41061=AXIS2_PLACEMENT_3D ( 'NONE', #37155, #54453, #2766 ) ;
#41086=CARTESIAN_POINT ( 'NONE',  ( -27.13182803479460858, 16.99370762638562127, 4.657392947539033656 ) ) ;
#41173=CARTESIAN_POINT ( 'NONE',  ( -23.23471500290295921, 19.24370688441070953, -4.657437592157546824 ) ) ;
#41206=CARTESIAN_POINT ( 'NONE',  ( -23.66772770479517618, 18.99370688441070953, 4.503109509781816122 ) ) ;
#41227=CARTESIAN_POINT ( 'NONE',  ( -24.54687786003638550, 18.44472464513734522, -4.546935035528026248 ) ) ;
#41236=EDGE_LOOP ( 'NONE', ( #16040, #32936, #26295, #37080 ) ) ;
#41243=VERTEX_POINT ( 'NONE', #18018 ) ;
#41257=MANIFOLD_SOLID_BREP ( 'Fillet5', #13160 ) ;
#41309=CARTESIAN_POINT ( 'NONE',  ( -23.66772770479517618, 18.99370688441070953, -4.657437592157546824 ) ) ;
#41320=CARTESIAN_POINT ( 'NONE',  ( -20.44406847140967187, 20.85488741058141571, -4.316516078624408337 ) ) ;
#41360=CARTESIAN_POINT ( 'NONE',  ( -28.92727693918987342, 15.95710471811680264, -4.722836279463598075 ) ) ;
#41515=CARTESIAN_POINT ( 'NONE',  ( -25.83279121425626812, 17.74370688441070953, 4.604227610039242968 ) ) ;
#41520=B_SPLINE_CURVE_WITH_KNOTS ( 'NONE', 3,
 ( #2450, #28561, #54976, #45890, #41360, #10957, #11537, #32809, #15242, #28855, #19482, #32556, #50127, #45592, #11238, #46415, #40796, #45324, #46154, #41878, #53838, #37647, #6435, #49859 ),
 .UNSPECIFIED., .F., .F.,
 ( 4, 1, 1, 1, 1, 2, 2, 1, 1, 1, 1, 1, 2, 2, 1, 1, 1, 4 ),
 ( 0.4483797419119410210, 0.4828560080424447176, 0.4914750745750705030, 0.4957846078413832847, 0.4979393744745396755, 0.4990167577911179264, 0.5000941411076962329, 0.5173322741729480256, 0.5862848064339559739, 0.7241898709559724256, 0.7414280040212243295, 0.7457375372875375552, 0.7478923039206943901, 0.7500470705538511140, 0.7586661370864771214, 0.7931424032169802629, 0.8620949354779869900, 1.000000000000000000 ),
 .UNSPECIFIED. ) ;
#41578=AXIS2_PLACEMENT_3D ( 'NONE', #10584, #14284, #27303 ) ;
#41588=CARTESIAN_POINT ( 'NONE',  ( -11.36804826722767103, 24.91136206679768605, -5.000000000000000888 ) ) ;
#41672=CARTESIAN_POINT ( 'NONE',  ( -46.55906441860520317, 5.863990010960497656, 5.000000000000000000 ) ) ;
#41681=CARTESIAN_POINT ( 'NONE',  ( -60.92294909528612834, 7.225036622302103417, -3.000000000000007105 ) ) ;
#41721=CARTESIAN_POINT ( 'NONE',  ( -27.56484202182514665, 16.74370688441070953, -4.657437592157546824 ) ) ;
#41766=EDGE_CURVE ( 'NONE', #460, #30957, #11260, .T. ) ;
#41787=CARTESIAN_POINT ( 'NONE',  ( -19.65677579747999459, 21.21320419402548296, -4.265613255889435074 ) ) ;
#41844=CARTESIAN_POINT ( 'NONE',  ( -46.28406441860931153, 5.387676038876692886, -5.000000000000000000 ) ) ;
#41870=DIRECTION ( 'NONE',  ( 0.8660254037844380415, 0.5000000000000011102, 0.000000000000000000 ) ) ;
#41877=ADVANCED_FACE ( 'NONE', ( #5115 ), #30677, .F. ) ;
#41878=CARTESIAN_POINT ( 'NONE',  ( -38.41289186640547371, 10.48058238645972651, -4.944624203975902077 ) ) ;
#41889=PLANE ( 'NONE',  #17998 ) ;
#41899=DIRECTION ( 'NONE',  ( -0.9335804264972041855, 0.3583679495452941066, 0.000000000000000000 ) ) ;
#41938=ORIENTED_EDGE ( 'NONE', *, *, #16749, .F. ) ;
#41968=DIRECTION ( 'NONE',  ( -0.8660254037844380415, -0.5000000000000011102, -0.000000000000000000 ) ) ;
#42015=AXIS2_PLACEMENT_3D ( 'NONE', #54751, #45672, #3375 ) ;
#42026=DIRECTION ( 'NONE',  ( -0.000000000000000000, -0.000000000000000000, -1.000000000000000000 ) ) ;
#42047=CARTESIAN_POINT ( 'NONE',  ( -55.84246788140315942, 5.810395100437911076, -3.000000000000007105 ) ) ;
#42076=AXIS2_PLACEMENT_3D ( 'NONE', #53468, #35895, #10314 ) ;
#42083=CARTESIAN_POINT ( 'NONE',  ( -27.56484202182514665, 16.74370688441070953, -4.657437592157546824 ) ) ;
#42088=CARTESIAN_POINT ( 'NONE',  ( -22.36868959911851462, 19.74370688441071309, 4.433756599430258127 ) ) ;
#42126=ORIENTED_EDGE ( 'NONE', *, *, #55203, .T. ) ;
#42156=CIRCLE ( 'NONE', #44023, 2.000000000000001776 ) ;
#42163=DIRECTION ( 'NONE',  ( 0.3535533905932752297, -0.6123724356957952475, -0.7071067811865462405 ) ) ;
#42170=DIRECTION ( 'NONE',  ( 0.5000000000000011102, -0.8660254037844380415, 0.000000000000000000 ) ) ;
#42205=CARTESIAN_POINT ( 'NONE',  ( -20.42601593468891963, 20.86531004751671148, 4.315323051534361021 ) ) ;
#42224=VERTEX_POINT ( 'NONE', #51877 ) ;
#42225=AXIS2_PLACEMENT_3D ( 'NONE', #40970, #49784, #28186 ) ;
#42235=ORIENTED_EDGE ( 'NONE', *, *, #14291, .T. ) ;
#42260=VERTEX_POINT ( 'NONE', #46798 ) ;
#42316=ORIENTED_EDGE ( 'NONE', *, *, #16790, .F. ) ;
#42331=EDGE_CURVE ( 'NONE', #51378, #55644, #36745, .T. ) ;
#42394=VERTEX_POINT ( 'NONE', #54585 ) ;
#42455=DIRECTION ( 'NONE',  ( -0.000000000000000000, -0.000000000000000000, -1.000000000000000000 ) ) ;
#42479=EDGE_CURVE ( 'NONE', #10688, #17567, #28205, .T. ) ;
#42550=CARTESIAN_POINT ( 'NONE',  ( -19.67731969574463236, 19.56551921504356883, 4.315409177132068841 ) ) ;
#42573=ORIENTED_EDGE ( 'NONE', *, *, #12836, .T. ) ;
#42641=PLANE ( 'NONE',  #39642 ) ;
#42681=DIRECTION ( 'NONE',  ( 1.007958083594381472E-15, -3.869188571150965639E-16, 1.000000000000000000 ) ) ;
#42683=CIRCLE ( 'NONE', #40870, 0.5000000000000004441 ) ;
#42707=CARTESIAN_POINT ( 'NONE',  ( -11.13054826722767032, 24.50000000000006395, -3.146497629411399100 ) ) ;
#42724=CARTESIAN_POINT ( 'NONE',  ( -24.53375310857961367, 18.49370688441070953, -4.657437592157546824 ) ) ;
#42743=CARTESIAN_POINT ( 'NONE',  ( -20.63663879154963965, 20.74370688441071664, 4.329123301634322907 ) ) ;
#42753=LINE ( 'NONE', #3858, #43207 ) ;
#42781=ORIENTED_EDGE ( 'NONE', *, *, #47577, .F. ) ;
#42817=DIRECTION ( 'NONE',  ( 0.3535533905932738974, -0.6123724356957929160, -0.7071067811865487940 ) ) ;
#42839=ORIENTED_EDGE ( 'NONE', *, *, #33593, .F. ) ;
#42845=EDGE_CURVE ( 'NONE', #21631, #16580, #40574, .T. ) ;
#42936=EDGE_LOOP ( 'NONE', ( #27653, #14395, #42839, #44260, #43576, #53346 ) ) ;
#42987=DIRECTION ( 'NONE',  ( 0.2113248654051873565, 0.7886751345948123104, 0.5773502691896265082 ) ) ;
#43001=CARTESIAN_POINT ( 'NONE',  ( -14.91381621359531984, 22.31572923274821463, -3.910276045922330912 ) ) ;
#43004=LINE ( 'NONE', #38767, #34077 ) ;
#43013=CARTESIAN_POINT ( 'NONE',  ( -25.92429756520238016, 17.40220053346460105, -4.407437592157546824 ) ) ;
#43035=LINE ( 'NONE', #55518, #19778 ) ;
#43102=DIRECTION ( 'NONE',  ( 0.3535533905932752297, -0.6123724356957952475, 0.7071067811865462405 ) ) ;
#43204=DIRECTION ( 'NONE',  ( -0.000000000000000000, -0.000000000000000000, -1.000000000000000000 ) ) ;
#43207=VECTOR ( 'NONE', #31104, 1000.000000000000000 ) ;
#43271=DIRECTION ( 'NONE',  ( 0.000000000000000000, 0.000000000000000000, 1.000000000000000000 ) ) ;
#43306=CARTESIAN_POINT ( 'NONE',  ( -12.97073463163625817, 23.43756790714967764, -3.644115791447929631 ) ) ;
#43325=DIRECTION ( 'NONE',  ( 0.9335804264972047406, -0.3583679495452924968, 0.000000000000000000 ) ) ;
#43335=CARTESIAN_POINT ( 'NONE',  ( -22.36868959911851462, 19.74370688441071309, 4.433756599430258127 ) ) ;
#43338=AXIS2_PLACEMENT_3D ( 'NONE', #50658, #46669, #11752 ) ;
#43346=CARTESIAN_POINT ( 'NONE',  ( -22.03063137938938354, 19.66613178766788295, -4.421226477812651545 ) ) ;
#43393=CARTESIAN_POINT ( 'NONE',  ( -24.40242990923838562, 16.83747556133229395, -4.580958211367532229 ) ) ;
#43447=CYLINDRICAL_SURFACE ( 'NONE', #37733, 0.5000000000000004441 ) ;
#43449=CARTESIAN_POINT ( 'NONE',  ( -20.72814514249575168, 20.40220053346460460, -4.657437592157546824 ) ) ;
#43487=VERTEX_POINT ( 'NONE', #44489 ) ;
#43576=ORIENTED_EDGE ( 'NONE', *, *, #31038, .T. ) ;
#43628=EDGE_LOOP ( 'NONE', ( #23722, #19301, #11138, #30232 ) ) ;
#43636=CARTESIAN_POINT ( 'NONE',  ( -20.63663879154963965, 20.74370688441071664, -4.657437592157546824 ) ) ;
#43647=CARTESIAN_POINT ( 'NONE',  ( -37.38198873126034272, 9.343723781475320678, -4.940473224498643567 ) ) ;
#43649=DIRECTION ( 'NONE',  ( 0.3583679495452941066, 0.9335804264972041855, -0.000000000000000000 ) ) ;
#43656=LINE ( 'NONE', #4238, #27312 ) ;
#43666=B_SPLINE_CURVE_WITH_KNOTS ( 'NONE', 3,
 ( #49084, #10186, #13607, #48536 ),
 .UNSPECIFIED., .F., .F.,
 ( 4, 4 ),
 ( 0.5868166818973559185, 0.6110328696463859233 ),
 .UNSPECIFIED. ) ;
#43681=DIRECTION ( 'NONE',  ( -0.000000000000000000, -0.000000000000000000, -1.000000000000000000 ) ) ;
#43691=DIRECTION ( 'NONE',  ( -0.000000000000000000, -0.000000000000000000, -1.000000000000000000 ) ) ;
#43714=CARTESIAN_POINT ( 'NONE',  ( -22.15441699824221899, 19.68629271404579484, -4.426028624882090590 ) ) ;
#43733=EDGE_CURVE ( 'NONE', #54076, #7274, #35044, .T. ) ;
#43799=CARTESIAN_POINT ( 'NONE',  ( -24.57312852195785524, 18.34675584111407787, 4.549864924635812713 ) ) ;
#43805=AXIS2_PLACEMENT_3D ( 'NONE', #31077, #1254, #53257 ) ;
#43812=PLANE ( 'NONE',  #36045 ) ;
#43815=LINE ( 'NONE', #22255, #21112 ) ;
#43827=ADVANCED_FACE ( 'NONE', ( #18038 ), #26846, .T. ) ;
#43839=LINE ( 'NONE', #40718, #15079 ) ;
#43883=CARTESIAN_POINT ( 'NONE',  ( -13.95518489968810627, 24.60124608745501007, -3.681743400992149695 ) ) ;
#43887=VECTOR ( 'NONE', #32706, 1000.000000000000000 ) ;
#43934=CARTESIAN_POINT ( 'NONE',  ( -45.77156441860525149, 4.499999999999981348, -5.000000000000000000 ) ) ;
#43956=VECTOR ( 'NONE', #38714, 1000.000000000000114 ) ;
#43974=ORIENTED_EDGE ( 'NONE', *, *, #33597, .T. ) ;
#44004=CARTESIAN_POINT ( 'NONE',  ( -21.96455284011576836, 19.88594039843075834, -4.412914656511901512 ) ) ;
#44023=AXIS2_PLACEMENT_3D ( 'NONE', #9510, #44692, #5265 ) ;
#44029=DIRECTION ( 'NONE',  ( -1.000000000000000000, 0.000000000000000000, 0.000000000000000000 ) ) ;
#44075=CARTESIAN_POINT ( 'NONE',  ( -60.74376512051347277, 7.691826835550698682, 2.999999999999993339 ) ) ;
#44080=FACE_OUTER_BOUND ( 'NONE', #27432, .T. ) ;
#44141=EDGE_CURVE ( 'NONE', #12681, #12998, #51206, .T. ) ;
#44151=ORIENTED_EDGE ( 'NONE', *, *, #17573, .T. ) ;
#44160=ORIENTED_EDGE ( 'NONE', *, *, #47577, .T. ) ;
#44183=CARTESIAN_POINT ( 'NONE',  ( -17.65907840528382522, 22.46280217494961562, -4.109392642200513812 ) ) ;
#44216=DIRECTION ( 'NONE',  ( -0.000000000000000000, -0.000000000000000000, 1.000000000000000000 ) ) ;
#44222=ORIENTED_EDGE ( 'NONE', *, *, #2855, .F. ) ;
#44238=CARTESIAN_POINT ( 'NONE',  ( -19.81260243149071698, 19.48741369114385691, -4.324310068654933836 ) ) ;
#44260=ORIENTED_EDGE ( 'NONE', *, *, #51737, .T. ) ;
#44302=DIRECTION ( 'NONE',  ( 0.2113248654051873565, 0.7886751345948121994, -0.5773502691896263972 ) ) ;
#44326=ORIENTED_EDGE ( 'NONE', *, *, #11093, .F. ) ;
#44334=( GEOMETRIC_REPRESENTATION_CONTEXT ( 3 ) GLOBAL_UNCERTAINTY_ASSIGNED_CONTEXT ( ( #46721 ) ) GLOBAL_UNIT_ASSIGNED_CONTEXT ( ( #30108, #5968, #5398 ) ) REPRESENTATION_CONTEXT ( 'NONE', 'WORKASPACE' ) );
#44338=EDGE_CURVE ( 'NONE', #3513, #34450, #50522, .T. ) ;
#44358=VERTEX_POINT ( 'NONE', #33209 ) ;
#44373=EDGE_CURVE ( 'NONE', #3752, #36925, #23819, .T. ) ;
#44400=ORIENTED_EDGE ( 'NONE', *, *, #53458, .F. ) ;
#44409=CARTESIAN_POINT ( 'NONE',  ( -25.25173380393689726, 18.07918053667318858, -4.578956201939200277 ) ) ;
#44436=ADVANCED_FACE ( 'NONE', ( #15234 ), #48458, .F. ) ;
#44439=CARTESIAN_POINT ( 'NONE',  ( -13.98444087813280490, 24.58435514042456660, -3.686392358618231668 ) ) ;
#44445=ORIENTED_EDGE ( 'NONE', *, *, #35247, .F. ) ;
#44457=CARTESIAN_POINT ( 'NONE',  ( -43.16120336687457382, 7.739143463467679673, 4.999999999999998224 ) ) ;
#44458=VERTEX_POINT ( 'NONE', #23471 ) ;
#44459=ORIENTED_EDGE ( 'NONE', *, *, #3718, .T. ) ;
#44488=CARTESIAN_POINT ( 'NONE',  ( -28.97056323743311523, 14.20006255460496547, -4.749095691681356257 ) ) ;
#44489=CARTESIAN_POINT ( 'NONE',  ( -20.63663879154963965, 20.74370688441071664, 4.329123301634322907 ) ) ;
#44545=ADVANCED_FACE ( 'NONE', ( #11529 ), #2691, .F. ) ;
#44549=FACE_OUTER_BOUND ( 'NONE', #5086, .T. ) ;
#44588=EDGE_LOOP ( 'NONE', ( #23903, #30975, #30288, #19028 ) ) ;
#44606=ADVANCED_FACE ( 'NONE', ( #28846 ), #32547, .F. ) ;
#44636=EDGE_CURVE ( 'NONE', #42224, #6825, #22353, .T. ) ;
#44650=EDGE_CURVE ( 'NONE', #54725, #30542, #15478, .T. ) ;
#44683=VERTEX_POINT ( 'NONE', #43013 ) ;
#44692=DIRECTION ( 'NONE',  ( -0.000000000000000000, -0.000000000000000000, -1.000000000000000000 ) ) ;
#44708=CIRCLE ( 'NONE', #38339, 2.000000000000002220 ) ;
#44710=ORIENTED_EDGE ( 'NONE', *, *, #31051, .T. ) ;
#44718=CARTESIAN_POINT ( 'NONE',  ( -18.63902545115410092, 21.89702948422484496, -4.188660131781243301 ) ) ;
#44723=CARTESIAN_POINT ( 'NONE',  ( -20.41971299214364421, 20.86894905309189596, -4.314906280119092941 ) ) ;
#44729=VECTOR ( 'NONE', #2628, 1000.000000000000000 ) ;
#44738=CARTESIAN_POINT ( 'NONE',  ( -28.48094711209952123, 16.21479336393476700, 4.707673465834044890 ) ) ;
#44781=CARTESIAN_POINT ( 'NONE',  ( -58.57533928340691887, 0.08623575067603483912, -3.000000000000007105 ) ) ;
#44827=ADVANCED_FACE ( 'NONE', ( #23615 ), #27611, .F. ) ;
#44841=DIRECTION ( 'NONE',  ( 0.000000000000000000, 0.000000000000000000, 1.000000000000000000 ) ) ;
#44843=PLANE ( 'NONE',  #34131 ) ;
#44918=LINE ( 'NONE', #44075, #31376 ) ;
#44982=CARTESIAN_POINT ( 'NONE',  ( -14.37032732058113993, 24.36156349900039331, 3.880826686532125258 ) ) ;
#44984=CARTESIAN_POINT ( 'NONE',  ( -23.29661994227107868, 19.01267450544941084, 4.488313114961025363 ) ) ;
#44987=CARTESIAN_POINT ( 'NONE',  ( -21.06965149344186372, 20.49370688441071664, 4.356723378946029790 ) ) ;
#45019=ORIENTED_EDGE ( 'NONE', *, *, #31051, .F. ) ;
#45030=CARTESIAN_POINT ( 'NONE',  ( -19.77061338776520216, 21.24370688441071664, -4.270683379717145733 ) ) ;
#45033=VERTEX_POINT ( 'NONE', #55974 ) ;
#45057=ORIENTED_EDGE ( 'NONE', *, *, #5695, .F. ) ;
#45087=VECTOR ( 'NONE', #16275, 1000.000000000000000 ) ;
#45090=CYLINDRICAL_SURFACE ( 'NONE', #34832, 0.5000000000000004441 ) ;
#45095=CARTESIAN_POINT ( 'NONE',  ( -20.63663870328428374, 20.74370693537071020, -4.329125112780540796 ) ) ;
#45175=EDGE_CURVE ( 'NONE', #44358, #2142, #9781, .T. ) ;
#45180=VERTEX_POINT ( 'NONE', #4555 ) ;
#45189=CARTESIAN_POINT ( 'NONE',  ( -49.27554558092695913, 2.476975532698160620, 5.000000000000000000 ) ) ;
#45209=EDGE_CURVE ( 'NONE', #12681, #25987, #12794, .T. ) ;
#45234=EDGE_LOOP ( 'NONE', ( #9051, #22597, #44326, #24231, #3709, #10397 ) ) ;
#45302=ORIENTED_EDGE ( 'NONE', *, *, #49320, .F. ) ;
#45324=CARTESIAN_POINT ( 'NONE',  ( -37.79788887702321176, 10.83565452793198425, -4.935543081462775206 ) ) ;
#45349=ORIENTED_EDGE ( 'NONE', *, *, #50318, .F. ) ;
#45418=CARTESIAN_POINT ( 'NONE',  ( -21.93567466420777379, 19.99370817364452790, -4.408991681665293427 ) ) ;
#45434=CARTESIAN_POINT ( 'NONE',  ( -27.22333567087903461, 16.65220053346459750, 4.407440554554201917 ) ) ;
#45435=ADVANCED_FACE ( 'NONE', ( #50523 ), #20701, .F. ) ;
#45542=AXIS2_PLACEMENT_3D ( 'NONE', #16394, #20685, #28920 ) ;
#45565=EDGE_CURVE ( 'NONE', #48717, #31783, #43656, .T. ) ;
#45571=EDGE_CURVE ( 'NONE', #9917, #39727, #31858, .T. ) ;
#45589=EDGE_CURVE ( 'NONE', #40704, #53976, #3924, .T. ) ;
#45592=CARTESIAN_POINT ( 'NONE',  ( -37.34829856057490360, 11.09522561815848007, -4.928657742077421133 ) ) ;
#45653=CARTESIAN_POINT ( 'NONE',  ( -11.64304826722810660, 25.38767603887884050, 5.000000000059520389 ) ) ;
#45672=DIRECTION ( 'NONE',  ( -0.2588190451025176864, -0.9659258262890692004, 0.000000000000000000 ) ) ;
#45686=AXIS2_PLACEMENT_3D ( 'NONE', #26181, #33847, #38692 ) ;
#45694=EDGE_LOOP ( 'NONE', ( #4195, #37133, #18236, #36714 ) ) ;
#45742=VECTOR ( 'NONE', #39731, 1000.000000000000114 ) ;
#45755=CARTESIAN_POINT ( 'NONE',  ( -25.85160320928759248, 17.67349956316208193, 4.606045228336897779 ) ) ;
#45764=ORIENTED_EDGE ( 'NONE', *, *, #45571, .T. ) ;
#45770=LINE ( 'NONE', #54294, #43887 ) ;
#45801=LINE ( 'NONE', #19955, #52755 ) ;
#45833=FACE_OUTER_BOUND ( 'NONE', #8943, .T. ) ;
#45864=CARTESIAN_POINT ( 'NONE',  ( -24.53375310857961367, 18.49370688441070953, 4.545578210335888159 ) ) ;
#45890=CARTESIAN_POINT ( 'NONE',  ( -28.72987205080237061, 16.07107648356668150, -4.716090232257376336 ) ) ;
#45956=DIRECTION ( 'NONE',  ( 1.000000000000000000, 0.000000000000000000, 0.000000000000000000 ) ) ;
#45981=EDGE_CURVE ( 'NONE', #682, #4092, #11819, .T. ) ;
#46026=FACE_OUTER_BOUND ( 'NONE', #35494, .T. ) ;
#46154=CARTESIAN_POINT ( 'NONE',  ( -37.92083312653435456, 10.76467263238142635, -4.937384707706697462 ) ) ;
#46181=CARTESIAN_POINT ( 'NONE',  ( -21.99342978027240392, 19.77817019059910564, 4.416855414988919648 ) ) ;
#46208=CARTESIAN_POINT ( 'NONE',  ( -61.21055533376208047, 7.871010810323351592, 2.999999999999993339 ) ) ;
#46324=VERTEX_POINT ( 'NONE', #34457 ) ;
#46342=B_SPLINE_CURVE_WITH_KNOTS ( 'NONE', 3,
 ( #9665, #31526, #22984, #5959 ),
 .UNSPECIFIED., .F., .F.,
 ( 4, 4 ),
 ( 0.000000000000000000, 0.0003538274413750522557 ),
 .UNSPECIFIED. ) ;
#46358=ORIENTED_EDGE ( 'NONE', *, *, #54169, .T. ) ;
#46372=LINE ( 'NONE', #50915, #50576 ) ;
#46383=CARTESIAN_POINT ( 'NONE',  ( -11.09304826722767956, 24.43504809471621186, -5.000000000000000888 ) ) ;
#46384=DIRECTION ( 'NONE',  ( 1.007958083594381669E-15, -3.869188571150966625E-16, 1.000000000000000000 ) ) ;
#46415=CARTESIAN_POINT ( 'NONE',  ( -37.71704171767562741, 10.88233165714454920, -4.934322635580619121 ) ) ;
#46438=CARTESIAN_POINT ( 'NONE',  ( -26.21622229497770817, 17.48042152905857449, -4.621141326338904065 ) ) ;
#46464=EDGE_CURVE ( 'NONE', #25142, #16114, #23080, .T. ) ;
#46508=AXIS2_PLACEMENT_3D ( 'NONE', #27113, #418, #4973 ) ;
#46535=B_SPLINE_CURVE_WITH_KNOTS ( 'NONE', 3,
 ( #2462, #50138, #32566, #15498 ),
 .UNSPECIFIED., .F., .F.,
 ( 4, 4 ),
 ( 0.3513510006676737740, 0.3765591803097264045 ),
 .UNSPECIFIED. ) ;
#46606=ORIENTED_EDGE ( 'NONE', *, *, #26825, .F. ) ;
#46610=FACE_OUTER_BOUND ( 'NONE', #1191, .T. ) ;
#46669=DIRECTION ( 'NONE',  ( 0.5000000000000011102, -0.8660254037844380415, 0.000000000000000000 ) ) ;
#46690=CARTESIAN_POINT ( 'NONE',  ( -20.69764258542294755, 20.51603762622108107, -4.338448882017707398 ) ) ;
#46712=DIRECTION ( 'NONE',  ( -0.9335804264972041855, 0.3583679495452941066, 1.079669255038093093E-15 ) ) ;
#46721=UNCERTAINTY_MEASURE_WITH_UNIT (LENGTH_MEASURE( 1.000000000000000082E-05 ), #30108, 'distance_accuracy_value', 'NONE');
#46729=ORIENTED_EDGE ( 'NONE', *, *, #45209, .F. ) ;
#46745=CARTESIAN_POINT ( 'NONE',  ( -19.95413052528122932, 21.13775321566489396, 4.283625658180314488 ) ) ;
#46798=CARTESIAN_POINT ( 'NONE',  ( -55.84246788140315942, 5.810395100437907523, 2.999999999999993339 ) ) ;
#46816=CARTESIAN_POINT ( 'NONE',  ( -22.95552628724609789, 17.67284575698099758, 4.512058519171590731 ) ) ;
#46842=VERTEX_POINT ( 'NONE', #53342 ) ;
#46884=ORIENTED_EDGE ( 'NONE', *, *, #46464, .T. ) ;
#46902=LINE ( 'NONE', #3158, #49277 ) ;
#46930=EDGE_LOOP ( 'NONE', ( #49134, #8266, #6117 ) ) ;
#46978=LINE ( 'NONE', #8642, #5983 ) ;
#47007=LINE ( 'NONE', #11786, #48521 ) ;
#47008=PLANE ( 'NONE',  #26692 ) ;
#47013=EDGE_LOOP ( 'NONE', ( #21647, #39092, #52286, #20503 ) ) ;
#47028=LINE ( 'NONE', #25435, #50249 ) ;
#47045=ORIENTED_EDGE ( 'NONE', *, *, #35247, .T. ) ;
#47085=CARTESIAN_POINT ( 'NONE',  ( -15.31839071495291726, 22.08214803548214533, 3.972478845913684165 ) ) ;
#47101=EDGE_CURVE ( 'NONE', #55644, #54555, #8296, .T. ) ;
#47110=CARTESIAN_POINT ( 'NONE',  ( -50.99228148001754590, 2.341865487272625668, -5.000000000000000000 ) ) ;
#47180=FACE_OUTER_BOUND ( 'NONE', #12965, .T. ) ;
#47220=CARTESIAN_POINT ( 'NONE',  ( -24.66083255426108423, 18.30077902615464680, 4.553899851047459535 ) ) ;
#47277=B_SPLINE_CURVE_WITH_KNOTS ( 'NONE', 3,
 ( #17743, #12055, #55794, #7832 ),
 .UNSPECIFIED., .F., .F.,
 ( 4, 4 ),
 ( 0.000000000000000000, 0.0003538863460371602767 ),
 .UNSPECIFIED. ) ;
#47312=ORIENTED_EDGE ( 'NONE', *, *, #4839, .F. ) ;
#47319=ORIENTED_EDGE ( 'NONE', *, *, #746, .T. ) ;
#47344=CARTESIAN_POINT ( 'NONE',  ( -23.66772770479517618, 18.99370688441070953, 4.503109509781816122 ) ) ;
#47356=CARTESIAN_POINT ( 'NONE',  ( -17.34288414376936416, 20.91330620938233409, 4.147373874202379795 ) ) ;
#47385=CARTESIAN_POINT ( 'NONE',  ( -23.23471500290295921, 19.24370688441070953, -4.657437592157546824 ) ) ;
#47399=ADVANCED_FACE ( 'NONE', ( #51229 ), #49622, .T. ) ;
#47402=EDGE_CURVE ( 'NONE', #12998, #11552, #44708, .T. ) ;
#47430=CARTESIAN_POINT ( 'NONE',  ( -23.29661890453421691, 19.01267837833611551, -4.488312987714206059 ) ) ;
#47445=VECTOR ( 'NONE', #3363, 1000.000000000000114 ) ;
#47465=DIRECTION ( 'NONE',  ( -0.000000000000000000, -0.000000000000000000, 1.000000000000000000 ) ) ;
#47504=CARTESIAN_POINT ( 'NONE',  ( -23.44702061269273230, 18.93456859731804087, -4.495868787147773382 ) ) ;
#47543=CARTESIAN_POINT ( 'NONE',  ( -13.20612570884338943, 23.30166480535930518, -3.681892822732769410 ) ) ;
#47577=EDGE_CURVE ( 'NONE', #4495, #46324, #43815, .T. ) ;
#47580=ORIENTED_EDGE ( 'NONE', *, *, #27250, .F. ) ;
#47585=CARTESIAN_POINT ( 'NONE',  ( -22.36868959911851462, 19.74370688441071309, -4.433759251830043269 ) ) ;
#47657=AXIS2_PLACEMENT_3D ( 'NONE', #24844, #42163, #34479 ) ;
#47731=DIRECTION ( 'NONE',  ( -0.9335804264972041855, 0.3583679495452941621, 0.000000000000000000 ) ) ;
#47759=ORIENTED_EDGE ( 'NONE', *, *, #45175, .T. ) ;
#47800=LINE ( 'NONE', #25941, #26800 ) ;
#47838=CARTESIAN_POINT ( 'NONE',  ( -15.34503691632512101, 22.06676384394702595, -3.956079653413159036 ) ) ;
#47866=B_SPLINE_CURVE_WITH_KNOTS ( 'NONE', 3,
 ( #8135, #17476, #50724, #55835, #29135, #7561, #24888, #3318, #8983, #26859, #48985, #48726, #13515, #5838, #14369, #30831, #26284, #43883, #44439, #39905, #5543, #31681, #9540, #39350, #31410, #48132, #10085, #985, #23160, #27398, #732, #44183, #44718, #18051 ),
 .UNSPECIFIED., .F., .F.,
 ( 4, 1, 1, 2, 2, 1, 1, 1, 1, 1, 2, 2, 1, 1, 1, 1, 1, 1, 2, 2, 1, 1, 1, 1, 1, 4 ),
 ( 0.000000000000000000, 0.02775256462266485064, 0.03469070577833101993, 0.03555797342278926160, 0.03577479033390380120, 0.03599160724501835468, 0.03642524106724729510, 0.03815977635616276537, 0.04162884693399369895, 0.05550512924531742637, 0.06244327040097930048, 0.06287690422320822703, 0.06331053804543715358, 0.06417780568989517320, 0.06591234097881149001, 0.06938141155664413751, 0.08325769386797447769, 0.1110102584906351164, 0.1248865408019652762, 0.1257538084464233652, 0.1266210760908814403, 0.1283556113797974241, 0.1318246819576294193, 0.1387628231132936596, 0.1665153877359508428, 0.2220205169812650703 ),
 .UNSPECIFIED. ) ;
#47922=DIRECTION ( 'NONE',  ( -0.2588190451025212946, -0.9659258262890680902, 0.000000000000000000 ) ) ;
#47925=CARTESIAN_POINT ( 'NONE',  ( -27.13182803479460858, 16.99370762638562127, 4.657392947539034544 ) ) ;
#47929=DIRECTION ( 'NONE',  ( -0.3583679495452941066, -0.9335804264972041855, 0.000000000000000000 ) ) ;
#47932=CARTESIAN_POINT ( 'NONE',  ( -30.80012389882216794, 13.14376521425323752, -4.804632802340537800 ) ) ;
#47985=CARTESIAN_POINT ( 'NONE',  ( -24.53375310857961367, 18.49370688441070953, 4.657440554554202805 ) ) ;
#47987=DIRECTION ( 'NONE',  ( -0.000000000000000000, -0.000000000000000000, 1.000000000000000000 ) ) ;
#47993=CARTESIAN_POINT ( 'NONE',  ( -22.36868959911851462, 19.74370688441071309, -4.433759251830043269 ) ) ;
#48024=VERTEX_POINT ( 'NONE', #53665 ) ;
#48064=ORIENTED_EDGE ( 'NONE', *, *, #16361, .F. ) ;
#48132=CARTESIAN_POINT ( 'NONE',  ( -16.10294711066915596, 23.36123499678980409, -3.956918830547554666 ) ) ;
#48168=EDGE_CURVE ( 'NONE', #2142, #54076, #19303, .T. ) ;
#48171=DIRECTION ( 'NONE',  ( 0.9659258262890682012, -0.2588190451025213501, 0.000000000000000000 ) ) ;
#48185=CARTESIAN_POINT ( 'NONE',  ( -16.45088425288988176, 21.42830258649871311, -4.066195520365398330 ) ) ;
#48193=DIRECTION ( 'NONE',  ( -1.007958083594381472E-15, 3.869188571150965639E-16, -1.000000000000000000 ) ) ;
#48202=VERTEX_POINT ( 'NONE', #34066 ) ;
#48312=LINE ( 'NONE', #35546, #33196 ) ;
#48358=ORIENTED_EDGE ( 'NONE', *, *, #24670, .F. ) ;
#48391=EDGE_CURVE ( 'NONE', #52053, #51242, #51453, .T. ) ;
#48399=ORIENTED_EDGE ( 'NONE', *, *, #5711, .T. ) ;
#48458=PLANE ( 'NONE',  #35045 ) ;
#48477=FACE_OUTER_BOUND ( 'NONE', #45234, .T. ) ;
#48480=CARTESIAN_POINT ( 'NONE',  ( -39.57685482548858147, 8.076517251137449449, -4.968603096491658100 ) ) ;
#48512=ORIENTED_EDGE ( 'NONE', *, *, #51737, .F. ) ;
#48518=VERTEX_POINT ( 'NONE', #18232 ) ;
#48521=VECTOR ( 'NONE', #33392, 1000.000000000000114 ) ;
#48536=CARTESIAN_POINT ( 'NONE',  ( -24.96676581047183063, 18.24370688441070953, 4.565775410814726598 ) ) ;
#48595=ORIENTED_EDGE ( 'NONE', *, *, #31565, .F. ) ;
#48611=VECTOR ( 'NONE', #13307, 1000.000000000000114 ) ;
#48641=CARTESIAN_POINT ( 'NONE',  ( -61.38973930853472893, 7.404220597074750998, -3.000000000000006661 ) ) ;
#48658=CIRCLE ( 'NONE', #24168, 0.5000000000000004441 ) ;
#48660=ORIENTED_EDGE ( 'NONE', *, *, #36328, .T. ) ;
#48717=VERTEX_POINT ( 'NONE', #32628 ) ;
#48726=CARTESIAN_POINT ( 'NONE',  ( -13.29351286303141322, 24.98326261593401298, -3.566503301129331227 ) ) ;
#48736=CARTESIAN_POINT ( 'NONE',  ( -19.77061338776520216, 21.24370688441071664, 4.270755533188014930 ) ) ;
#48748=DIRECTION ( 'NONE',  ( -0.7886751345948130876, 0.2113248654051844977, -0.5773502691896263972 ) ) ;
#48837=DIRECTION ( 'NONE',  ( 0.3535533905932752297, -0.6123724356957952475, 0.7071067811865462405 ) ) ;
#48842=( LENGTH_UNIT ( ) NAMED_UNIT ( * ) SI_UNIT ( .MILLI., .METRE. ) );
#48876=CARTESIAN_POINT ( 'NONE',  ( -24.62525945952572215, 18.15220053346460105, -4.657437592157546824 ) ) ;
#48932=CARTESIAN_POINT ( 'NONE',  ( -22.36868959911851462, 19.74370688441071309, -4.433759251830043269 ) ) ;
#48985=CARTESIAN_POINT ( 'NONE',  ( -13.09680306462247046, 25.09683307099765770, -3.525414222879889259 ) ) ;
#49013=VERTEX_POINT ( 'NONE', #45095 ) ;
#49084=CARTESIAN_POINT ( 'NONE',  ( -25.83279121425626812, 17.74370688441070953, 4.604227610039242968 ) ) ;
#49092=DIRECTION ( 'NONE',  ( 0.8660254037844380415, 0.5000000000000011102, 0.000000000000000000 ) ) ;
#49096=CARTESIAN_POINT ( 'NONE',  ( -24.96676581047183063, 18.24370688441070953, -4.657437592157546824 ) ) ;
#49130=EDGE_CURVE ( 'NONE', #48024, #44458, #55535, .T. ) ;
#49134=ORIENTED_EDGE ( 'NONE', *, *, #31038, .F. ) ;
#49164=CARTESIAN_POINT ( 'NONE',  ( -61.38973930853472893, 7.404220597074750998, -3.000000000000006661 ) ) ;
#49222=CARTESIAN_POINT ( 'NONE',  ( -21.93567689722629765, 19.99370688441071309, 4.408989160011352659 ) ) ;
#49256=CARTESIAN_POINT ( 'NONE',  ( -23.23471098716119698, 19.24370920290025566, -4.480780584866845828 ) ) ;
#49277=VECTOR ( 'NONE', #55393, 1000.000000000000114 ) ;
#49320=EDGE_CURVE ( 'NONE', #3513, #52053, #14147, .T. ) ;
#49321=DIRECTION ( 'NONE',  ( 0.3583679495452941066, 0.9335804264972041855, -0.000000000000000000 ) ) ;
#49490=CARTESIAN_POINT ( 'NONE',  ( -19.39860431275361918, 21.26603824944624677, 4.250162336167266020 ) ) ;
#49513=EDGE_CURVE ( 'NONE', #4495, #40047, #8073, .T. ) ;
#49520=CARTESIAN_POINT ( 'NONE',  ( -11.88464697727586916, 25.79667171432705430, 3.467463535836658561 ) ) ;
#49622=( BOUNDED_SURFACE ( )  B_SPLINE_SURFACE ( 2, 3, ( 
 ( #11762, #41844, #2944, #23986 ),
 ( #20277, #29079, #41588, #46383 ),
 ( #3528, #12348, #32777, #37061 ) ),
 .UNSPECIFIED., .F., .F., .F. ) 
 B_SPLINE_SURFACE_WITH_KNOTS ( ( 3, 3 ),
 ( 4, 4 ),
 ( 0.000000000000000000, 1.000000000000000000 ),
 ( 0.0004250000000000007895, 0.002075000000000026476 ),
 .UNSPECIFIED. ) 
 GEOMETRIC_REPRESENTATION_ITEM ( )  RATIONAL_B_SPLINE_SURFACE ( (
 ( 1.000000000000000000, 1.000000000000000000, 1.000000000000000000, 1.000000000000000000),
 ( 0.7071067811865484609, 0.7071067811865484609, 0.7071067811865475727, 0.7071067811865475727),
 ( 1.000000000000000000, 1.000000000000000000, 1.000000000000000000, 1.000000000000000000) ) ) 
 REPRESENTATION_ITEM ( '' )  SURFACE ( )  );
#49624=CARTESIAN_POINT ( 'NONE',  ( -56.20083583094844926, 4.876814673940706335, 2.999999999999993339 ) ) ;
#49674=FACE_OUTER_BOUND ( 'NONE', #39194, .T. ) ;
#49677=DIRECTION ( 'NONE',  ( 0.5000000000000011102, -0.8660254037844380415, 0.000000000000000000 ) ) ;
#49729=VECTOR ( 'NONE', #47987, 1000.000000000000000 ) ;
#49783=ORIENTED_EDGE ( 'NONE', *, *, #19738, .F. ) ;
#49784=DIRECTION ( 'NONE',  ( 0.000000000000000000, -0.000000000000000000, -1.000000000000000000 ) ) ;
#49825=DIRECTION ( 'NONE',  ( -0.000000000000000000, -0.000000000000000000, -1.000000000000000000 ) ) ;
#49845=CARTESIAN_POINT ( 'NONE',  ( -26.54131626755147977, 17.33463975416308500, 4.634068379122165737 ) ) ;
#49859=CARTESIAN_POINT ( 'NONE',  ( -46.52156441860571334, 5.799038105676371124, -5.000000000000000000 ) ) ;
#49891=DIRECTION ( 'NONE',  ( -0.000000000000000000, -0.000000000000000000, -1.000000000000000000 ) ) ;
#49965=ORIENTED_EDGE ( 'NONE', *, *, #26007, .F. ) ;
#49968=ADVANCED_FACE ( 'NONE', ( #21033 ), #55687, .F. ) ;
#49969=AXIS2_PLACEMENT_3D ( 'NONE', #9063, #43681, #35204 ) ;
#49975=VERTEX_POINT ( 'NONE', #3452 ) ;
#49982=CARTESIAN_POINT ( 'NONE',  ( -23.52058642966956370, 18.95428049856751329, 4.498258486333376993 ) ) ;
#49999=ADVANCED_FACE ( 'NONE', ( #26706 ), #18177, .T. ) ;
#50039=( NAMED_UNIT ( * ) SI_UNIT ( $, .STERADIAN. ) SOLID_ANGLE_UNIT ( ) );
#50050=CARTESIAN_POINT ( 'NONE',  ( -24.53375310857961367, 18.49370688441070953, -4.657437592157546824 ) ) ;
#50089=DIRECTION ( 'NONE',  ( 0.9335804264972044075, -0.3583679495452936070, 0.000000000000000000 ) ) ;
#50127=CARTESIAN_POINT ( 'NONE',  ( -35.40880390783866716, 12.21499337800758234, -4.897373001089857958 ) ) ;
#50138=CARTESIAN_POINT ( 'NONE',  ( -23.95238608277258407, 18.82935929325833513, -4.517660165671053996 ) ) ;
#50202=DIRECTION ( 'NONE',  ( -0.2588190451025212946, -0.9659258262890680902, 0.000000000000000000 ) ) ;
#50245=AXIS2_PLACEMENT_3D ( 'NONE', #35764, #22974, #14199 ) ;
#50249=VECTOR ( 'NONE', #55829, 1000.000000000000000 ) ;
#50309=CARTESIAN_POINT ( 'NONE',  ( -23.66772770479517618, 18.99370688441070953, -4.503111145262439052 ) ) ;
#50318=EDGE_CURVE ( 'NONE', #39727, #38353, #38814, .T. ) ;
#50319=ORIENTED_EDGE ( 'NONE', *, *, #30721, .T. ) ;
#50341=CARTESIAN_POINT ( 'NONE',  ( -27.22333567087903461, 16.65220053346459750, -4.657437592157546824 ) ) ;
#50343=PRESENTATION_STYLE_ASSIGNMENT (( #53239 ) ) ;
#50367=LINE ( 'NONE', #19716, #45087 ) ;
#50372=B_SPLINE_CURVE_WITH_KNOTS ( 'NONE', 3,
 ( #8905, #26208, #39254, #51496 ),
 .UNSPECIFIED., .F., .F.,
 ( 4, 4 ),
 ( 3.934737272476643706E-05, 0.0004522109935135529301 ),
 .UNSPECIFIED. ) ;
#50394=CARTESIAN_POINT ( 'NONE',  ( -22.03895444026947104, 19.66185708466576187, 4.421688969255889390 ) ) ;
#50425=EDGE_CURVE ( 'NONE', #27945, #51378, #54625, .T. ) ;
#50426=EDGE_LOOP ( 'NONE', ( #26186, #6535, #31567, #49965, #6832 ) ) ;
#50522=LINE ( 'NONE', #24651, #27781 ) ;
#50523=FACE_OUTER_BOUND ( 'NONE', #46930, .T. ) ;
#50544=DIRECTION ( 'NONE',  ( -0.9335804264972041855, 0.3583679495452941621, 0.000000000000000000 ) ) ;
#50563=EDGE_CURVE ( 'NONE', #54555, #30542, #56073, .T. ) ;
#50576=VECTOR ( 'NONE', #12018, 1000.000000000000000 ) ;
#50630=CARTESIAN_POINT ( 'NONE',  ( -61.70068505767309830, 8.059153983834628221, -3.000000000000000000 ) ) ;
#50650=DIRECTION ( 'NONE',  ( 0.3583679495452925523, 0.9335804264972047406, 0.000000000000000000 ) ) ;
#50658=CARTESIAN_POINT ( 'NONE',  ( -50.02554558092695913, 3.776013638374817294, 5.000000000000000000 ) ) ;
#50674=ADVANCED_FACE ( 'NONE', ( #38159 ), #3529, .T. ) ;
#50679=EDGE_CURVE ( 'NONE', #46842, #19985, #46978, .T. ) ;
#50724=CARTESIAN_POINT ( 'NONE',  ( -12.16389985764536519, 25.63544498867374344, -3.297528153982450583 ) ) ;
#50768=CARTESIAN_POINT ( 'NONE',  ( -20.95581447963227717, 20.46320434849166148, -4.352198852488014857 ) ) ;
#50794=ORIENTED_EDGE ( 'NONE', *, *, #54169, .F. ) ;
#50823=EDGE_CURVE ( 'NONE', #54087, #9690, #21700, .T. ) ;
#50846=EDGE_LOOP ( 'NONE', ( #34818, #8963, #54722, #2186 ) ) ;
#50858=VERTEX_POINT ( 'NONE', #50309 ) ;
#50870=CARTESIAN_POINT ( 'NONE',  ( -25.92429756520238016, 17.40220053346460105, -4.657437592157546824 ) ) ;
#50895=EDGE_CURVE ( 'NONE', #52748, #35993, #24210, .T. ) ;
#50915=CARTESIAN_POINT ( 'NONE',  ( -23.23471500290295921, 19.24370688441070953, 4.657440554554202805 ) ) ;
#50941=CARTESIAN_POINT ( 'NONE',  ( -15.35456184398319657, 22.06126462439962310, -3.957089338018470404 ) ) ;
#51061=ORIENTED_EDGE ( 'NONE', *, *, #50823, .T. ) ;
#51206=LINE ( 'NONE', #29660, #24120 ) ;
#51229=FACE_OUTER_BOUND ( 'NONE', #8555, .T. ) ;
#51235=ORIENTED_EDGE ( 'NONE', *, *, #25260, .T. ) ;
#51242=VERTEX_POINT ( 'NONE', #9115 ) ;
#51246=CARTESIAN_POINT ( 'NONE',  ( -12.42987990997295711, 23.74983052629447045, -3.542935327883032226 ) ) ;
#51248=FACE_OUTER_BOUND ( 'NONE', #3464, .T. ) ;
#51261=FACE_OUTER_BOUND ( 'NONE', #22575, .T. ) ;
#51279=DIRECTION ( 'NONE',  ( -0.000000000000000000, -0.000000000000000000, -1.000000000000000000 ) ) ;
#51345=ORIENTED_EDGE ( 'NONE', *, *, #15082, .T. ) ;
#51349=CARTESIAN_POINT ( 'NONE',  ( -20.84197899872282633, 20.43270222331197061, -4.347644189607536624 ) ) ;
#51378=VERTEX_POINT ( 'NONE', #45418 ) ;
#51437=ORIENTED_EDGE ( 'NONE', *, *, #35015, .F. ) ;
#51453=B_SPLINE_CURVE_WITH_KNOTS ( 'NONE', 3,
 ( #23459, #44457, #5560, #27719, #6154, #54114, #2121, #32535, #1840, #19168, #32261, #10936, #44738, #14385, #53539 ),
 .UNSPECIFIED., .F., .F.,
 ( 4, 1, 1, 1, 1, 1, 2, 2, 1, 1, 4 ),
 ( 0.000000000000000000, 0.2700693087945782445, 0.4051039631918675887, 0.4726212903905119833, 0.4895006221901730958, 0.4979402880900037909, 0.4989952463274826555, 0.5000502045649615201, 0.5021601210399194715, 0.5063799539898351521, 0.5401386175891612629 ),
 .UNSPECIFIED. ) ;
#51462=EDGE_CURVE ( 'NONE', #16114, #33400, #12188, .T. ) ;
#51496=CARTESIAN_POINT ( 'NONE',  ( -25.85160216376510434, 17.67350346510513148, -4.606045122360801436 ) ) ;
#51533=EDGE_LOOP ( 'NONE', ( #5561, #18494, #1551, #46884 ) ) ;
#51570=CARTESIAN_POINT ( 'NONE',  ( -20.46240439165153191, 20.84430116209394868, 4.317727107778031481 ) ) ;
#51602=CARTESIAN_POINT ( 'NONE',  ( -27.56484202182514665, 16.74370688441070953, -4.657437592157546824 ) ) ;
#51608=CARTESIAN_POINT ( 'NONE',  ( -11.13054826722768098, 24.50000000000005684, 3.000000000000000444 ) ) ;
#51617=ADVANCED_FACE ( 'NONE', ( #12753 ), #30071, .F. ) ;
#51668=CARTESIAN_POINT ( 'NONE',  ( -61.38973930853472183, 7.404220597074748333, 2.999999999999993339 ) ) ;
#51698=PLANE ( 'NONE',  #3952 ) ;
#51718=ORIENTED_EDGE ( 'NONE', *, *, #33597, .F. ) ;
#51722=ORIENTED_EDGE ( 'NONE', *, *, #31222, .F. ) ;
#51729=PLANE ( 'NONE',  #9421 ) ;
#51737=EDGE_CURVE ( 'NONE', #14093, #54725, #15813, .T. ) ;
#51744=DIRECTION ( 'NONE',  ( 0.9335804264972041855, -0.3583679495452941066, 0.000000000000000000 ) ) ;
#51809=CYLINDRICAL_SURFACE ( 'NONE', #7026, 2.000000000000001332 ) ;
#51877=CARTESIAN_POINT ( 'NONE',  ( -56.38001980572109062, 4.410024460692103077, -3.000000000000007105 ) ) ;
#51898=DIRECTION ( 'NONE',  ( 0.000000000000000000, -0.000000000000000000, -1.000000000000000000 ) ) ;
#51913=ORIENTED_EDGE ( 'NONE', *, *, #37432, .F. ) ;
#51941=DIRECTION ( 'NONE',  ( 0.9335804264972044075, -0.3583679495452936070, 0.000000000000000000 ) ) ;
#52022=CARTESIAN_POINT ( 'NONE',  ( -23.23471500290295921, 19.24370688441070953, -4.657437592157546824 ) ) ;
#52053=VERTEX_POINT ( 'NONE', #37003 ) ;
#52078=CARTESIAN_POINT ( 'NONE',  ( -12.12997044929294965, 23.92298333415059375, -3.477585481046854721 ) ) ;
#52107=AXIS2_PLACEMENT_3D ( 'NONE', #10197, #44841, #35477 ) ;
#52151=EDGE_CURVE ( 'NONE', #35896, #34812, #310, .T. ) ;
#52170=VECTOR ( 'NONE', #7567, 999.9999999999998863 ) ;
#52181=PLANE ( 'NONE',  #30162 ) ;
#52184=EDGE_CURVE ( 'NONE', #15174, #37067, #5976, .T. ) ;
#52191=SHAPE_DEFINITION_REPRESENTATION ( #40961, #24540 ) ;
#52195=CARTESIAN_POINT ( 'NONE',  ( -19.06545585621813999, 19.91877896750159138, 4.274096488885640532 ) ) ;
#52275=VECTOR ( 'NONE', #22028, 1000.000000000000000 ) ;
#52280=ORIENTED_EDGE ( 'NONE', *, *, #1552, .F. ) ;
#52286=ORIENTED_EDGE ( 'NONE', *, *, #33111, .F. ) ;
#52394=DIRECTION ( 'NONE',  ( 0.3535533905932738974, -0.6123724356957929160, 0.7071067811865487940 ) ) ;
#52441=EDGE_CURVE ( 'NONE', #40396, #21504, #237, .T. ) ;
#52478=CARTESIAN_POINT ( 'NONE',  ( -25.83279121425626812, 17.74370688441070953, -4.657437592157546824 ) ) ;
#52529=FILL_AREA_STYLE ('',( #841 ) ) ;
#52607=CARTESIAN_POINT ( 'NONE',  ( -23.66772770479517618, 18.99370688441070953, -4.503111145262439052 ) ) ;
#52613=FACE_OUTER_BOUND ( 'NONE', #963, .T. ) ;
#52620=ORIENTED_EDGE ( 'NONE', *, *, #36974, .F. ) ;
#52711=ADVANCED_FACE ( 'NONE', ( #21778 ), #16976, .F. ) ;
#52726=CARTESIAN_POINT ( 'NONE',  ( -15.46945900645201100, 21.99492871671912653, -3.969181436210386771 ) ) ;
#52748=VERTEX_POINT ( 'NONE', #7592 ) ;
#52755=VECTOR ( 'NONE', #11988, 1000.000000000000000 ) ;
#52792=DIRECTION ( 'NONE',  ( 1.007958083594381669E-15, -3.869188571150966625E-16, 1.000000000000000000 ) ) ;
#53002=CARTESIAN_POINT ( 'NONE',  ( -55.84246788140315942, 5.810395100437911076, 5.000000000000000000 ) ) ;
#53012=CARTESIAN_POINT ( 'NONE',  ( -27.22333567087903461, 16.65220053346459750, -4.407437592157545048 ) ) ;
#53026=CARTESIAN_POINT ( 'NONE',  ( -44.29771021218551397, 5.350930122822688872, -5.000000000000003553 ) ) ;
#53051=ORIENTED_EDGE ( 'NONE', *, *, #29439, .F. ) ;
#53101=VECTOR ( 'NONE', #1459, 999.9999999999998863 ) ;
#53124=ADVANCED_FACE ( 'NONE', ( #29099 ), #4123, .F. ) ;
#53177=DIRECTION ( 'NONE',  ( 0.000000000000000000, -0.000000000000000000, -1.000000000000000000 ) ) ;
#53239=SURFACE_STYLE_USAGE ( .BOTH. , #18575 ) ;
#53257=DIRECTION ( 'NONE',  ( -0.2588190451025212946, -0.9659258262890680902, 0.000000000000000000 ) ) ;
#53342=CARTESIAN_POINT ( 'NONE',  ( -25.92429756520238016, 17.40220053346459750, 4.407440554554201917 ) ) ;
#53346=ORIENTED_EDGE ( 'NONE', *, *, #47101, .F. ) ;
#53391=CARTESIAN_POINT ( 'NONE',  ( -24.83619032682412353, 18.20871928901600256, 4.561852666301203563 ) ) ;
#53392=ORIENTED_EDGE ( 'NONE', *, *, #17293, .T. ) ;
#53458=EDGE_CURVE ( 'NONE', #55644, #607, #7729, .T. ) ;
#53468=CARTESIAN_POINT ( 'NONE',  ( -63.00984630926863161, 1.788483511016180305, 2.999999999999993339 ) ) ;
#53505=CARTESIAN_POINT ( 'NONE',  ( -26.55142373434009073, 17.32880420549185985, -4.634472827760601099 ) ) ;
#53536=ADVANCED_FACE ( 'NONE', ( #12577 ), #3749, .F. ) ;
#53539=CARTESIAN_POINT ( 'NONE',  ( -27.56460882755735398, 16.74384151918395247, 4.673983433494172779 ) ) ;
#53550=EDGE_CURVE ( 'NONE', #36925, #16114, #16055, .T. ) ;
#53597=ORIENTED_EDGE ( 'NONE', *, *, #45565, .F. ) ;
#53665=CARTESIAN_POINT ( 'NONE',  ( -23.32622135384906770, 18.90220053346460460, -4.407437592157546824 ) ) ;
#53672=PLANE ( 'NONE',  #13696 ) ;
#53675=ORIENTED_EDGE ( 'NONE', *, *, #10469, .F. ) ;
#53709=DIRECTION ( 'NONE',  ( 0.000000000000000000, -0.000000000000000000, -1.000000000000000000 ) ) ;
#53719=VECTOR ( 'NONE', #54754, 1000.000000000000000 ) ;
#53814=ORIENTED_EDGE ( 'NONE', *, *, #37251, .F. ) ;
#53838=CARTESIAN_POINT ( 'NONE',  ( -39.69590723381624997, 9.739833118710683024, -4.961795781091632662 ) ) ;
#53856=DIRECTION ( 'NONE',  ( -1.000000000000000000, 0.000000000000000000, 0.000000000000000000 ) ) ;
#53873=ADVANCED_FACE ( 'NONE', ( #16386 ), #34559, .F. ) ;
#53934=VERTEX_POINT ( 'NONE', #51608 ) ;
#53952=ORIENTED_EDGE ( 'NONE', *, *, #13492, .T. ) ;
#53954=B_SPLINE_CURVE_WITH_KNOTS ( 'NONE', 3,
 ( #46438, #20638, #7556, #29733 ),
 .UNSPECIFIED., .F., .F.,
 ( 4, 4 ),
 ( 0.0003023226855361189165, 0.0003536700609687475679 ),
 .UNSPECIFIED. ) ;
#53976=VERTEX_POINT ( 'NONE', #29770 ) ;
#54009=ORIENTED_EDGE ( 'NONE', *, *, #38351, .T. ) ;
#54014=CARTESIAN_POINT ( 'NONE',  ( -24.57312748012714820, 18.34675972927921350, -4.549864808573585329 ) ) ;
#54076=VERTEX_POINT ( 'NONE', #9868 ) ;
#54087=VERTEX_POINT ( 'NONE', #53012 ) ;
#54114=CARTESIAN_POINT ( 'NONE',  ( -29.54997447658847776, 15.59759012727598915, 4.743609536075380717 ) ) ;
#54116=ORIENTED_EDGE ( 'NONE', *, *, #33811, .F. ) ;
#54136=ORIENTED_EDGE ( 'NONE', *, *, #16749, .T. ) ;
#54161=AXIS2_PLACEMENT_3D ( 'NONE', #27107, #5807, #52394 ) ;
#54169=EDGE_CURVE ( 'NONE', #9690, #34711, #41520, .T. ) ;
#54174=DIRECTION ( 'NONE',  ( -0.2588190451025212946, -0.9659258262890680902, 0.000000000000000000 ) ) ;
#54179=ORIENTED_EDGE ( 'NONE', *, *, #44636, .T. ) ;
#54230=ADVANCED_FACE ( 'NONE', ( #8375 ), #51809, .T. ) ;
#54294=CARTESIAN_POINT ( 'NONE',  ( -61.52150108290046404, 8.525944197083212828, -5.000000000000000000 ) ) ;
#54342=CARTESIAN_POINT ( 'NONE',  ( -63.56784591066751489, 8.775889882925216767, 3.000000000000000000 ) ) ;
#54359=CARTESIAN_POINT ( 'NONE',  ( -61.70068505767309830, 8.059153983834628221, 3.000000000000000000 ) ) ;
#54366=ADVANCED_FACE ( 'NONE', ( #40153 ), #31916, .F. ) ;
#54372=CARTESIAN_POINT ( 'NONE',  ( -23.95239534612751697, 18.82935394505787130, 4.517658012124546651 ) ) ;
#54425=ORIENTED_EDGE ( 'NONE', *, *, #47101, .T. ) ;
#54426=CARTESIAN_POINT ( 'NONE',  ( -22.02718324817240969, 19.65220053346460816, -4.657437592157546824 ) ) ;
#54453=DIRECTION ( 'NONE',  ( 0.3535533905932752297, -0.6123724356957952475, 0.7071067811865462405 ) ) ;
#54474=ORIENTED_EDGE ( 'NONE', *, *, #49130, .T. ) ;
#54499=DIRECTION ( 'NONE',  ( -0.2588190451025176864, -0.9659258262890692004, 0.000000000000000000 ) ) ;
#54555=VERTEX_POINT ( 'NONE', #2637 ) ;
#54585=CARTESIAN_POINT ( 'NONE',  ( -24.83619454210204580, 18.20872041849631984, -4.561852789702152577 ) ) ;
#54606=ORIENTED_EDGE ( 'NONE', *, *, #746, .F. ) ;
#54625=B_SPLINE_CURVE_WITH_KNOTS ( 'NONE', 3,
 ( #22334, #27407, #8991, #31418 ),
 .UNSPECIFIED., .F., .F.,
 ( 4, 4 ),
 ( 0.2710609481134873544, 0.2986749355271498541 ),
 .UNSPECIFIED. ) ;
#54684=CARTESIAN_POINT ( 'NONE',  ( -20.41408287047329750, 20.87219960535384544, 4.314533580056656881 ) ) ;
#54722=ORIENTED_EDGE ( 'NONE', *, *, #29222, .F. ) ;
#54725=VERTEX_POINT ( 'NONE', #13968 ) ;
#54742=B_SPLINE_CURVE_WITH_KNOTS ( 'NONE', 3,
 ( #42743, #33412, #7555, #51570, #33669, #55530, #42205, #54684, #20886, #3848, #46745, #33965 ),
 .UNSPECIFIED., .F., .F.,
 ( 4, 1, 1, 2, 2, 1, 1, 4 ),
 ( 0.7429994551377537837, 0.7471935825069564441, 0.7492906461915580518, 0.7498149121127086758, 0.7500770450732842098, 0.7503391780338596329, 0.7513877098761616580, 0.7597759646145790802 ),
 .UNSPECIFIED. ) ;
#54751=CARTESIAN_POINT ( 'NONE',  ( -22.36868959911851462, 19.74370688441071309, -4.657437592157546824 ) ) ;
#54754=DIRECTION ( 'NONE',  ( -0.000000000000000000, -0.000000000000000000, 1.000000000000000000 ) ) ;
#54758=CARTESIAN_POINT ( 'NONE',  ( -49.27554558092695913, 2.476975532698160620, -5.000000000000000000 ) ) ;
#54797=ADVANCED_FACE ( 'NONE', ( #40378 ), #39250, .F. ) ;
#54838=VECTOR ( 'NONE', #31660, 1000.000000000000114 ) ;
#54853=CIRCLE ( 'NONE', #34040, 0.5000000000000004441 ) ;
#54860=VERTEX_POINT ( 'NONE', #32140 ) ;
#54871=DIRECTION ( 'NONE',  ( -0.000000000000000000, -0.000000000000000000, 1.000000000000000000 ) ) ;
#54886=DIRECTION ( 'NONE',  ( 0.3583679495452941066, 0.9335804264972041855, -0.000000000000000000 ) ) ;
#54913=B_SPLINE_CURVE_WITH_KNOTS ( 'NONE', 3,
 ( #43934, #53026, #22081, #48480, #9879, #13304, #43647, #30630, #5058, #9600, #9293, #21798, #39117, #47932, #39957, #44488, #35423, #26616, #193, #26924, #1042, #27182, #26087, #39703, #43393, #17843, #780, #14140, #4759, #44238, #39413, #4490, #35712, #5338, #13565, #30876, #17541, #48185, #22387, #18099, #52726, #13833, #4399, #50941, #47838, #17427, #43001, #21712, #25679, #56079, #30528, #39024, #47543, #8658, #3540, #20597, #43306, #8941, #51246, #38171, #55221, #38458, #12363, #55785, #52078, #26243, #42707, #17166 ),
 .UNSPECIFIED., .F., .F.,
 ( 4, 1, 1, 1, 1, 1, 1, 2, 2, 1, 1, 1, 1, 1, 1, 1, 1, 2, 2, 1, 1, 1, 1, 1, 1, 1, 1, 2, 2, 1, 1, 1, 1, 1, 1, 1, 2, 2, 1, 1, 1, 1, 1, 1, 2, 2, 1, 1, 1, 2, 2, 1, 1, 4 ),
 ( 0.000000000000000000, 0.1249999999999907296, 0.1874999999999860945, 0.2187499999999835687, 0.2343749999999822642, 0.2421874999999815703, 0.2460937499999812095, 0.2480468749999808209, 0.2499999999999804323, 0.3749999999999575340, 0.4374999999999463207, 0.4687499999999407141, 0.4843749999999379385, 0.4921874999999364952, 0.4960937499999357736, 0.4980468749999352740, 0.4990234374999349964, 0.4995117187499349409, 0.4999999999999348299, 0.6249999999999096278, 0.6874999999998971933, 0.7187499999998909761, 0.7343749999998877565, 0.7421874999998862021, 0.7460937499998856470, 0.7480468749998852029, 0.7490234374998852029, 0.7495117187498852029, 0.7499999999998853140, 0.8124999999999193978, 0.8437499999999364952, 0.8593749999999450440, 0.8671874999999493738, 0.8710937499999514833, 0.8730468749999525935, 0.8740234374999530376, 0.8745117187499533706, 0.8749999999999535927, 0.9062499999999694689, 0.9218749999999774625, 0.9296874999999815703, 0.9335937499999836797, 0.9355468749999849010, 0.9365234374999853451, 0.9370117187499856781, 0.9374999999999860112, 0.9531249999999898970, 0.9609374999999920064, 0.9619140624999922284, 0.9624023437499923395, 0.9628906249999924505, 0.9648437499999927836, 0.9687499999999936717, 1.000000000000000000 ),
 .UNSPECIFIED. ) ;
#54942=ORIENTED_EDGE ( 'NONE', *, *, #9859, .F. ) ;
#54964=DIRECTION ( 'NONE',  ( -1.000000000000000000, 0.000000000000000000, 0.000000000000000000 ) ) ;
#54967=ORIENTED_EDGE ( 'NONE', *, *, #39714, .F. ) ;
#54976=CARTESIAN_POINT ( 'NONE',  ( -28.11332263830040645, 16.42704145284338324, -4.694618095106484645 ) ) ;
#55067=DIRECTION ( 'NONE',  ( -0.8660254037844380415, -0.5000000000000011102, -0.000000000000000000 ) ) ;
#55074=PLANE ( 'NONE',  #13302 ) ;
#55075=ORIENTED_EDGE ( 'NONE', *, *, #14552, .T. ) ;
#55104=ORIENTED_EDGE ( 'NONE', *, *, #32393, .T. ) ;
#55117=ORIENTED_EDGE ( 'NONE', *, *, #52441, .T. ) ;
#55126=EDGE_CURVE ( 'NONE', #27103, #27671, #34633, .T. ) ;
#55171=ORIENTED_EDGE ( 'NONE', *, *, #4839, .T. ) ;
#55203=EDGE_CURVE ( 'NONE', #4092, #51378, #3, .T. ) ;
#55221=CARTESIAN_POINT ( 'NONE',  ( -12.32171488119139546, 23.81227963477840248, -3.519960964911045931 ) ) ;
#55223=ORIENTED_EDGE ( 'NONE', *, *, #12515, .T. ) ;
#55262=EDGE_CURVE ( 'NONE', #10688, #42394, #5964, .T. ) ;
#55274=EDGE_LOOP ( 'NONE', ( #18917, #47312, #2604, #3426 ) ) ;
#55315=CARTESIAN_POINT ( 'NONE',  ( -11.13054826722768098, 24.50000000000005684, 3.000000000000000444 ) ) ;
#55333=ADVANCED_FACE ( 'NONE', ( #40308 ), #41889, .T. ) ;
#55393=DIRECTION ( 'NONE',  ( 0.3583679495452941066, 0.9335804264972041855, -0.000000000000000000 ) ) ;
#55400=ORIENTED_EDGE ( 'NONE', *, *, #42331, .T. ) ;
#55409=VECTOR ( 'NONE', #40814, 1000.000000000000114 ) ;
#55423=DIRECTION ( 'NONE',  ( 0.000000000000000000, 0.000000000000000000, -1.000000000000000000 ) ) ;
#55433=AXIS2_PLACEMENT_3D ( 'NONE', #33476, #38015, #42817 ) ;
#55445=ORIENTED_EDGE ( 'NONE', *, *, #33272, .F. ) ;
#55450=B_SPLINE_CURVE_WITH_KNOTS ( 'NONE', 3,
 ( #47585, #8706, #132, #49256 ),
 .UNSPECIFIED., .F., .F.,
 ( 4, 4 ),
 ( 0.3121479134361153651, 0.3384768704940201989 ),
 .UNSPECIFIED. ) ;
#55454=EDGE_CURVE ( 'NONE', #34450, #36925, #43035, .T. ) ;
#55518=CARTESIAN_POINT ( 'NONE',  ( -49.27554558092695913, 2.476975532698160620, 5.000000000000000000 ) ) ;
#55530=CARTESIAN_POINT ( 'NONE',  ( -20.42824791815107943, 20.86402141126400167, 4.315470560068479955 ) ) ;
#55535=LINE ( 'NONE', #3005, #14925 ) ;
#55584=ORIENTED_EDGE ( 'NONE', *, *, #11163, .F. ) ;
#55644=VERTEX_POINT ( 'NONE', #25370 ) ;
#55659=DIRECTION ( 'NONE',  ( 1.000000000000000000, 0.000000000000000000, -8.673617379884027583E-16 ) ) ;
#55662=EDGE_CURVE ( 'NONE', #44458, #44358, #3449, .T. ) ;
#55682=CARTESIAN_POINT ( 'NONE',  ( -25.83278826518980154, 17.74370858705499288, -4.604226652742015702 ) ) ;
#55687=PLANE ( 'NONE',  #6817 ) ;
#55745=CARTESIAN_POINT ( 'NONE',  ( -23.39689275304487737, 18.96061820135890130, -4.493364476181771039 ) ) ;
#55785=CARTESIAN_POINT ( 'NONE',  ( -12.24874546236494588, 23.85440854838047642, -3.504140126263841637 ) ) ;
#55794=CARTESIAN_POINT ( 'NONE',  ( -19.54294029912370334, 21.18270206417091828, 4.260498045019209812 ) ) ;
#55810=CARTESIAN_POINT ( 'NONE',  ( -45.77156441860526570, 4.499999999999973355, 5.000000000000000000 ) ) ;
#55829=DIRECTION ( 'NONE',  ( 0.000000000000000000, 0.000000000000000000, -1.000000000000000000 ) ) ;
#55835=CARTESIAN_POINT ( 'NONE',  ( -12.81737946304616926, 25.25815836258565383, -3.463348302191213257 ) ) ;
#55937=VECTOR ( 'NONE', #21796, 1000.000000000000000 ) ;
#55974=CARTESIAN_POINT ( 'NONE',  ( -23.29661994227107868, 19.01267450544941084, 4.488313114961025363 ) ) ;
#55999=DIRECTION ( 'NONE',  ( 0.3535533905932752297, -0.6123724356957952475, -0.7071067811865462405 ) ) ;
#56027=LINE ( 'NONE', #52022, #43956 ) ;
#56031=FACE_BOUND ( 'NONE', #50846, .T. ) ;
#56073=B_SPLINE_CURVE_WITH_KNOTS ( 'NONE', 3,
 ( #28241, #2412, #50394, #19156 ),
 .UNSPECIFIED., .F., .F.,
 ( 4, 4 ),
 ( 0.0002402743607020580493, 0.0002683764075209547190 ),
 .UNSPECIFIED. ) ;
#56077=B_SPLINE_CURVE_WITH_KNOTS ( 'NONE', 3,
 ( #37075, #36505, #49845, #15471 ),
 .UNSPECIFIED., .F., .F.,
 ( 4, 4 ),
 ( 0.5515979657728906638, 0.5753284354475328710 ),
 .UNSPECIFIED. ) ;
#56079=CARTESIAN_POINT ( 'NONE',  ( -13.44167438888726984, 23.16567071152870838, -3.718480911511438336 ) ) ;
#56080=ADVANCED_FACE ( 'NONE', ( #40088 ), #1743, .F. ) ;
#56163=APPLICATION_CONTEXT ( 'automotive_design' ) ;
#56169=LINE ( 'NONE', #26335, #5085 ) ;
#56217=CARTESIAN_POINT ( 'NONE',  ( -49.27554558092695913, 2.476975532698160620, -5.000000000000000000 ) ) ;
#56230=CARTESIAN_POINT ( 'NONE',  ( -22.26155278157260042, 19.71499966066964760, -4.429874095009547652 ) ) ;
#56236=DIRECTION ( 'NONE',  ( -1.000000000000000000, 0.000000000000000000, 0.000000000000000000 ) ) ;
ENDSEC;
END-ISO-10303-21;
